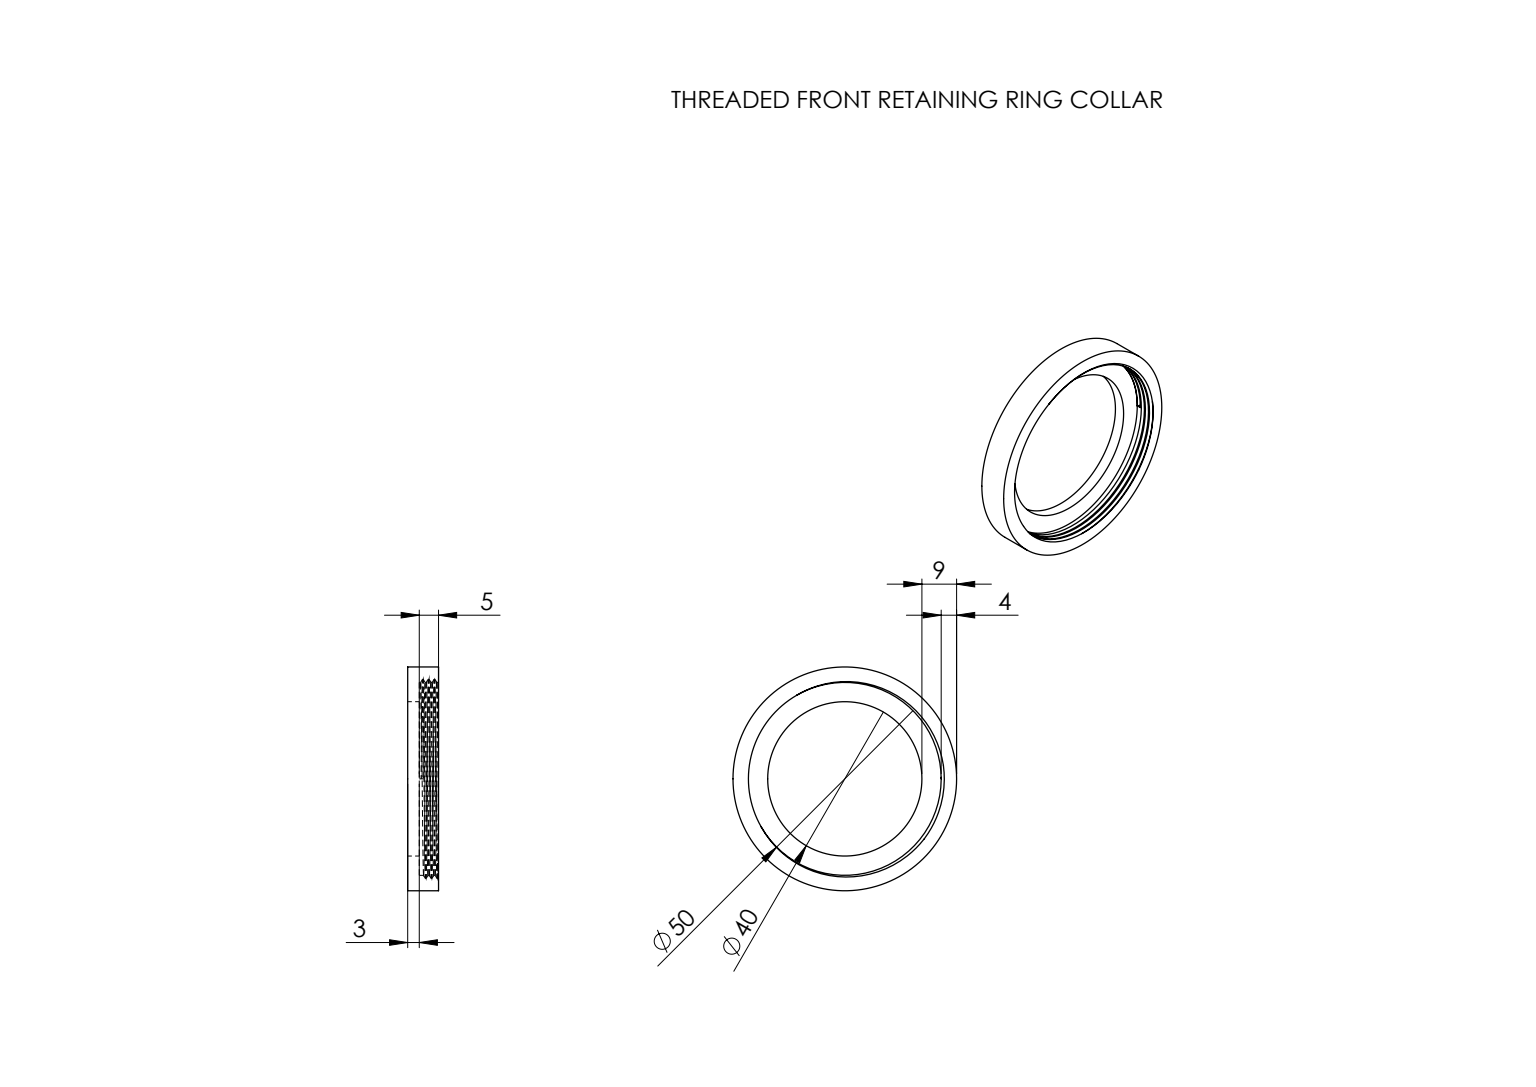
ISO-10303-21;
HEADER;
FILE_DESCRIPTION (('STEP AP214'),
    '1' );
FILE_NAME ('Threaded Front Retaining Ring Collar.step',
    '2026-10-22T10:02:39',
    ( '' ),
    ( '' ),
    'SwSTEP 2.0',
    'SolidWorks 2026',
    '' );
FILE_SCHEMA (( 'AUTOMOTIVE_DESIGN' ));
ENDSEC;

DATA;
#16=CARTESIAN_POINT ( 'NONE',  ( -75.12500000204838102, 44.30836144126050158, -25.81189881249999374 ) ) ;
#42=CARTESIAN_POINT ( 'NONE',  ( -78.87500000204838102, 65.69163855873949842, 25.81189881250000440 ) ) ;
#54=CARTESIAN_POINT ( 'NONE',  ( -72.59375000204838102, 55.00000000000000000, 25.81189881249999729 ) ) ;
#55=EDGE_CURVE ( 'NONE', #2377, #9420, #11722, .T. ) ;
#67=DIRECTION ( 'NONE',  ( -1.000000000000000000, 0.000000000000000000, 0.000000000000000000 ) ) ;
#76=CARTESIAN_POINT ( 'NONE',  ( -72.50000000204839523, 29.18810118750000981, 10.69163855873950020 ) ) ;
#83=ORIENTED_EDGE ( 'NONE', *, *, #6664, .F. ) ;
#110=CARTESIAN_POINT ( 'NONE',  ( -77.75000000204839523, 65.69163855873948421, -25.81189881250000084 ) ) ;
#117=CARTESIAN_POINT ( 'NONE',  ( -78.50000000409677625, 80.00000000000000000, -1.530808498934191324E-15 ) ) ;
#125=AXIS2_PLACEMENT_3D ( 'NONE', #5377, #67, #9915 ) ;
#129=CARTESIAN_POINT ( 'NONE',  ( -79.34375000000000000, 65.35533905932734910, 24.99999999999997158 ) ) ;
#131=VERTEX_POINT ( 'NONE', #8809 ) ;
#166=CARTESIAN_POINT ( 'NONE',  ( -74.56250000204839523, 80.81189881250001861, 10.69163855873948599 ) ) ;
#176=( BOUNDED_CURVE ( )  B_SPLINE_CURVE ( 2, ( #5683, #4899, #11229, #6928, #8370, #6645, #9381, #4776, #5808 ),
 .UNSPECIFIED., .F., .T. ) 
 B_SPLINE_CURVE_WITH_KNOTS ( ( 3, 2, 2, 2, 3 ),
 ( 0.3333333333333335924, 0.3541666666666669627, 0.3750000000000003331, 0.3958333333333336479, 0.4166666666666670182 ),
 .UNSPECIFIED. ) 
 CURVE ( )  GEOMETRIC_REPRESENTATION_ITEM ( )  RATIONAL_B_SPLINE_CURVE ( ( 0.9999999999999990008, 0.9238795325112877377, 1.000000000000000000, 0.9238795325112867385, 1.000000000000000000, 0.9238795325112867385, 1.000000000000000000, 0.9238795325112855172, 1.000000000000001110 ) ) 
 REPRESENTATION_ITEM ( '' )  );
#177=CARTESIAN_POINT ( 'NONE',  ( -75.00000000000000000, 63.49954157109033304, -24.30489545910771909 ) ) ;
#219=CARTESIAN_POINT ( 'NONE',  ( -78.31250000000000000, 72.67766952966368876, -17.67766952966368876 ) ) ;
#225=ORIENTED_EDGE ( 'NONE', *, *, #438, .T. ) ;
#231=CARTESIAN_POINT ( 'NONE',  ( -71.59560441781462714, 80.81189881250000440, 6.916273779317701376 ) ) ;
#238=CARTESIAN_POINT ( 'NONE',  ( -78.87500000204839523, 65.69163855873949842, 25.81189881250000084 ) ) ;
#239=CARTESIAN_POINT ( 'NONE',  ( -75.00000000000002842, 78.51577914341699227, 8.706246595591601078 ) ) ;
#275=CARTESIAN_POINT ( 'NONE',  ( -79.53125000000000000, 80.00000000000001421, 10.35533905932737397 ) ) ;
#288=CARTESIAN_POINT ( 'NONE',  ( -77.93750000204838102, 44.30836144126050158, -25.81189881249999374 ) ) ;
#297=CARTESIAN_POINT ( 'NONE',  ( -75.00000000000000000, 78.71525423744449768, -9.017306879578036671 ) ) ;
#304=CARTESIAN_POINT ( 'NONE',  ( -72.21875000409676204, 65.35533905932737753, 24.99999999999999645 ) ) ;
#307=EDGE_CURVE ( 'NONE', #8475, #1715, #7669, .T. ) ;
#335=CARTESIAN_POINT ( 'NONE',  ( -75.96875000000000000, 30.00000000000001421, 10.35533905932739174 ) ) ;
#347=CARTESIAN_POINT ( 'NONE',  ( -76.81250000204839523, 29.18810118750000981, 10.69163855873950020 ) ) ;
#354=FACE_BOUND ( 'NONE', #1822, .T. ) ;
#361=CARTESIAN_POINT ( 'NONE',  ( -72.12500000409677625, 55.00000000000000000, 24.99999999999999645 ) ) ;
#363=FACE_OUTER_BOUND ( 'NONE', #3792, .T. ) ;
#370=CIRCLE ( 'NONE', #6328, 25.00000000000000355 ) ;
#383=ORIENTED_EDGE ( 'NONE', *, *, #4826, .F. ) ;
#393=VECTOR ( 'NONE', #8335, 1000.000000000000000 ) ;
#397=CARTESIAN_POINT ( 'NONE',  ( -77.37500000000000000, 30.00000000000000355, 4.592425496802573578E-15 ) ) ;
#400=LINE ( 'NONE', #10690, #6493 ) ;
#401=AXIS2_PLACEMENT_3D ( 'NONE', #2687, #9038, #3756 ) ;
#402=CARTESIAN_POINT ( 'NONE',  ( -75.00000000000000000, 55.00000000000000000, 25.00000000000000355 ) ) ;
#410=CARTESIAN_POINT ( 'NONE',  ( -79.06250000204840944, 80.81189881250001861, -10.69163855873949132 ) ) ;
#417=CARTESIAN_POINT ( 'NONE',  ( -79.34375000204839523, 73.25176868561975141, -18.25176868561974430 ) ) ;
#418=PLANE ( 'NONE',  #9121 ) ;
#420=ORIENTED_EDGE ( 'NONE', *, *, #2126, .F. ) ;
#422=CARTESIAN_POINT ( 'NONE',  ( -72.03125000409679046, 44.64466094067262958, 25.00000000000001066 ) ) ;
#438=EDGE_CURVE ( 'NONE', #9864, #879, #4301, .T. ) ;
#451=CARTESIAN_POINT ( 'NONE',  ( -78.87500000000002842, 30.00000000000003553, 4.592425496802568845E-15 ) ) ;
#456=CARTESIAN_POINT ( 'NONE',  ( -72.78125000000002842, 30.00000000000000355, -10.35533905932738108 ) ) ;
#459=DIRECTION ( 'NONE',  ( 1.000000000000000000, -0.000000000000000000, -0.000000000000000000 ) ) ;
#468=CARTESIAN_POINT ( 'NONE',  ( -75.31250000204839523, 29.18810118750000981, 10.69163855873950020 ) ) ;
#475=DIRECTION ( 'NONE',  ( 0.000000000000000000, 0.000000000000000000, 1.000000000000000000 ) ) ;
#478=( GEOMETRIC_REPRESENTATION_CONTEXT ( 3 ) GLOBAL_UNCERTAINTY_ASSIGNED_CONTEXT ( ( #4789 ) ) GLOBAL_UNIT_ASSIGNED_CONTEXT ( ( #10005, #10508, #11461 ) ) REPRESENTATION_CONTEXT ( 'NONE', 'WORKASPACE' ) );
#480=CARTESIAN_POINT ( 'NONE',  ( -79.25000000000000000, 55.00000000000000000, 24.99999999999999645 ) ) ;
#487=CARTESIAN_POINT ( 'NONE',  ( -78.12500000409677625, 55.00000000000000000, 24.99999999999999645 ) ) ;
#510=CARTESIAN_POINT ( 'NONE',  ( -74.18750000000000000, 37.32233047033631124, -17.67766952966368166 ) ) ;
#515=CYLINDRICAL_SURFACE ( 'NONE', #11802, 29.00000000000000355 ) ;
#525=CARTESIAN_POINT ( 'NONE',  ( -76.62500000204839523, 29.18810118750000626, -10.69163855873949309 ) ) ;
#529=CARTESIAN_POINT ( 'NONE',  ( -75.49999999999972999, 55.00000000002793854, -24.99999999999999645 ) ) ;
#532=CARTESIAN_POINT ( 'NONE',  ( -77.84375000204839523, 73.25176868561975141, -18.25176868561974430 ) ) ;
#544=CARTESIAN_POINT ( 'NONE',  ( -78.50000000409677625, 80.00000000000000000, -1.530808498934191324E-15 ) ) ;
#550=CARTESIAN_POINT ( 'NONE',  ( -78.03125000204839523, 36.74823131438024859, -18.25176868561973720 ) ) ;
#557=CARTESIAN_POINT ( 'NONE',  ( -75.00000000000004263, 38.53867536077979139, -19.88773376194887987 ) ) ;
#559=ORIENTED_EDGE ( 'NONE', *, *, #6186, .F. ) ;
#566=AXIS2_PLACEMENT_3D ( 'NONE', #8644, #10369, #4811 ) ;
#568=CARTESIAN_POINT ( 'NONE',  ( -73.25000000000000000, 55.00000000000000000, 24.99999999999999645 ) ) ;
#582=CARTESIAN_POINT ( 'NONE',  ( -73.15625000204839523, 73.25176868561975141, -18.25176868561974430 ) ) ;
#601=ORIENTED_EDGE ( 'NONE', *, *, #9027, .F. ) ;
#614=CARTESIAN_POINT ( 'NONE',  ( -76.62500000204839523, 29.18810118750000626, -10.69163855873949309 ) ) ;
#618=CARTESIAN_POINT ( 'NONE',  ( -74.99999999999997158, 37.75762616273102168, -19.19216994046665903 ) ) ;
#627=CARTESIAN_POINT ( 'NONE',  ( -73.90625000000001421, 65.35533905932737753, -24.99999999999999645 ) ) ;
#629=ADVANCED_FACE ( 'NONE', ( #7359 ), #4594, .T. ) ;
#638=DIRECTION ( 'NONE',  ( -1.000000000000000000, 0.000000000000000000, 0.000000000000000000 ) ) ;
#641=CARTESIAN_POINT ( 'NONE',  ( -74.93750000204839523, 44.30836144126050158, -25.81189881249999374 ) ) ;
#649=CARTESIAN_POINT ( 'NONE',  ( -75.87500000204838102, 65.69163855873949842, 25.81189881250000084 ) ) ;
#667=CARTESIAN_POINT ( 'NONE',  ( -74.84375000204839523, 55.00000000000000000, -25.81189881249999729 ) ) ;
#674=CARTESIAN_POINT ( 'NONE',  ( -74.99999999999998579, 36.28446816562487243, -17.71219965803775764 ) ) ;
#675=ORIENTED_EDGE ( 'NONE', *, *, #799, .F. ) ;
#685=CARTESIAN_POINT ( 'NONE',  ( -71.95822497812569907, 74.53807824654330716, 16.15905817987090032 ) ) ;
#689=CARTESIAN_POINT ( 'NONE',  ( -80.00000000000000000, 55.00000000000000000, -24.99999999999999645 ) ) ;
#693=VECTOR ( 'NONE', #6124, 1000.000000000000000 ) ;
#694=CARTESIAN_POINT ( 'NONE',  ( -74.99999999999998579, 39.36515909056227258, -20.53791299142420712 ) ) ;
#705=CARTESIAN_POINT ( 'NONE',  ( -75.03125000204838102, 55.00000000000000000, -25.81189881249999729 ) ) ;
#725=CARTESIAN_POINT ( 'NONE',  ( -78.50000000204840944, 44.30836144126053000, 25.81189881250000795 ) ) ;
#728=CARTESIAN_POINT ( 'NONE',  ( -76.62500000409677625, 55.00000000000000000, 24.99999999999999645 ) ) ;
#730=CARTESIAN_POINT ( 'NONE',  ( -75.00000000000001421, 29.55542218757419803, 0.4186910811744771199 ) ) ;
#742=CARTESIAN_POINT ( 'NONE',  ( -72.40625000204838102, 29.18810118750000271, 4.741568889096522788E-15 ) ) ;
#748=VECTOR ( 'NONE', #2550, 1000.000000000000000 ) ;
#763=B_SPLINE_CURVE_WITH_KNOTS ( 'NONE', 3,
 ( #2945, #11252, #6612, #5710, #177, #2885, #3718, #10057, #10117, #6673, #7383, #6488, #10302, #1917, #5585, #3779, #4804, #9408, #8461, #10239, #1201, #8516, #297, #9170, #4743, #9347, #4678, #1016, #7622, #1855, #6554, #1135, #8329, #7448, #10183, #239, #9282, #1319, #3124, #9702 ),
 .UNSPECIFIED., .F., .F.,
 ( 4, 2, 2, 2, 2, 2, 2, 2, 2, 2, 2, 2, 2, 2, 2, 2, 2, 2, 2, 4 ),
 ( 2.472710646779110686E-15, 0.003130555644250782206, 0.006261111288499070747, 0.009391666932747358421, 0.01095694475487150529, 0.01252222257699565390, 0.01565277822124398407, 0.01721805604336814829, 0.01878333386549230904, 0.02504444515398900756, 0.02660972297611319259, 0.02817500079823737763, 0.03130555644248574770, 0.03443611208673411084, 0.03600138990885830281, 0.03756666773098249479, 0.04382777901947923493, 0.04539305684160341997, 0.04695833466372760501, 0.05008889030797599590 ),
 .UNSPECIFIED. ) ;
#769=CARTESIAN_POINT ( 'NONE',  ( -74.84375000204839523, 73.25176868561975141, -18.25176868561974430 ) ) ;
#784=CARTESIAN_POINT ( 'NONE',  ( -76.06250000204840944, 80.81189881250001861, -10.69163855873949132 ) ) ;
#790=CARTESIAN_POINT ( 'NONE',  ( -75.00000000000000000, 34.71505921034813724, 14.90932262158721500 ) ) ;
#799=EDGE_CURVE ( 'NONE', #1715, #10833, #3542, .T. ) ;
#801=CARTESIAN_POINT ( 'NONE',  ( -72.68750000204839523, 44.30836144126053000, 25.81189881250000795 ) ) ;
#823=CARTESIAN_POINT ( 'NONE',  ( -83.00000000000000000, 55.00000000000000000, 20.00000000000000355 ) ) ;
#832=CARTESIAN_POINT ( 'NONE',  ( -76.53125000204839523, 36.74823131438024859, -18.25176868561973720 ) ) ;
#838=CARTESIAN_POINT ( 'NONE',  ( -75.59375000409679046, 80.00000000000001421, -10.35533905932737753 ) ) ;
#855=CARTESIAN_POINT ( 'NONE',  ( -75.03125000204838102, 55.00000000000000000, -25.81189881249999729 ) ) ;
#870=ORIENTED_EDGE ( 'NONE', *, *, #7718, .F. ) ;
#879=VERTEX_POINT ( 'NONE', #5025 ) ;
#891=CARTESIAN_POINT ( 'NONE',  ( -76.62500000204838102, 29.18810118750000626, -10.69163855873949132 ) ) ;
#897=CARTESIAN_POINT ( 'NONE',  ( -76.62500000409677625, 55.00000000000000000, 24.99999999999999645 ) ) ;
#898=CARTESIAN_POINT ( 'NONE',  ( -75.50000000409677625, 80.00000000000000000, -1.530808498934191324E-15 ) ) ;
#906=ORIENTED_EDGE ( 'NONE', *, *, #8266, .F. ) ;
#912=MANIFOLD_SOLID_BREP ( 'Cavity1', #11314 ) ;
#913=EDGE_CURVE ( 'NONE', #1407, #8886, #6011, .T. ) ;
#914=CARTESIAN_POINT ( 'NONE',  ( -74.18750000204838102, 44.30836144126053000, 25.81189881250000795 ) ) ;
#924=AXIS2_PLACEMENT_3D ( 'NONE', #3401, #7187, #2623 ) ;
#936=AXIS2_PLACEMENT_3D ( 'NONE', #10985, #6463, #1890 ) ;
#945=CARTESIAN_POINT ( 'NONE',  ( -76.71875000204839523, 36.74823131438024859, -18.25176868561973720 ) ) ;
#953=CARTESIAN_POINT ( 'NONE',  ( -75.00000000000000000, 55.00000000000000000, 29.00000000000000355 ) ) ;
#958=DIRECTION ( 'NONE',  ( 0.000000000000000000, 0.000000000000000000, -1.000000000000000000 ) ) ;
#963=CARTESIAN_POINT ( 'NONE',  ( -73.25000000204839523, 65.69163855873948421, -25.81189881250000440 ) ) ;
#981=CARTESIAN_POINT ( 'NONE',  ( -72.31250000204839523, 29.18810118750000626, -10.69163855873949309 ) ) ;
#1006=CARTESIAN_POINT ( 'NONE',  ( -83.00000000000000000, 55.00000000000000000, 29.00000000000000355 ) ) ;
#1009=CARTESIAN_POINT ( 'NONE',  ( -76.43750000204838102, 65.69163855873948421, -25.81189881250000440 ) ) ;
#1014=CARTESIAN_POINT ( 'NONE',  ( -78.96875000204839523, 80.81189881250000440, -1.580522963032174394E-15 ) ) ;
#1016=CARTESIAN_POINT ( 'NONE',  ( -75.00000000000001421, 80.17654715216286831, -1.959916203278639024 ) ) ;
#1020=CARTESIAN_POINT ( 'NONE',  ( -71.56250000204838102, 80.81189881250001861, -10.69163855873949132 ) ) ;
#1067=CARTESIAN_POINT ( 'NONE',  ( -73.25000000204838102, 80.81189881250001861, -10.69163855873949132 ) ) ;
#1080=VECTOR ( 'NONE', #11683, 1000.000000000000000 ) ;
#1082=CARTESIAN_POINT ( 'NONE',  ( -76.53125000409677625, 44.64466094067262958, 25.00000000000001066 ) ) ;
#1104=CARTESIAN_POINT ( 'NONE',  ( -80.00000000000000000, 55.00000000000000000, -24.99999999999999645 ) ) ;
#1115=CARTESIAN_POINT ( 'NONE',  ( -79.62500000000000000, 80.00000000000000000, -1.530808498934191324E-15 ) ) ;
#1127=CARTESIAN_POINT ( 'NONE',  ( -73.71875000204839523, 36.74823131438024859, -18.25176868561973720 ) ) ;
#1134=CARTESIAN_POINT ( 'NONE',  ( -79.53125000204838102, 55.00000000000000000, -25.81189881249999729 ) ) ;
#1135=CARTESIAN_POINT ( 'NONE',  ( -75.00000000000001421, 80.11351121041060708, 2.705448568323045144 ) ) ;
#1140=CARTESIAN_POINT ( 'NONE',  ( -73.53125000409676204, 44.64466094067262958, 25.00000000000001066 ) ) ;
#1178=CARTESIAN_POINT ( 'NONE',  ( -78.21875000000001421, 80.00000000000001421, -10.35533905932737753 ) ) ;
#1194=CARTESIAN_POINT ( 'NONE',  ( -79.15625000204839523, 73.25176868561975141, -18.25176868561974430 ) ) ;
#1201=CARTESIAN_POINT ( 'NONE',  ( -75.00000000000000000, 78.13883143010173171, -10.47133000126702917 ) ) ;
#1205=CARTESIAN_POINT ( 'NONE',  ( -74.18750000409677625, 72.67766952966368876, -17.67766952966368876 ) ) ;
#1223=CARTESIAN_POINT ( 'NONE',  ( -78.12500000000004263, 79.99999999999992895, -1.530808498934187183E-15 ) ) ;
#1228=CARTESIAN_POINT ( 'NONE',  ( -78.50000000000000000, 55.00000000000000000, -24.99999999999999645 ) ) ;
#1231=CARTESIAN_POINT ( 'NONE',  ( -75.00000000000001421, 76.68791387293471473, 12.43520775219157315 ) ) ;
#1233=CARTESIAN_POINT ( 'NONE',  ( -79.06250000000001421, 37.32233047033631124, 17.67766952966369232 ) ) ;
#1234=CARTESIAN_POINT ( 'NONE',  ( -74.99999999999997158, 42.18634379380805655, -22.42280631998790597 ) ) ;
#1237=FACE_OUTER_BOUND ( 'NONE', #7141, .T. ) ;
#1246=CARTESIAN_POINT ( 'NONE',  ( -77.18750000204839523, 65.69163855873949842, 25.81189881250000440 ) ) ;
#1260=CARTESIAN_POINT ( 'NONE',  ( -74.65625000409679046, 30.00000000000000355, -10.35533905932738108 ) ) ;
#1273=ORIENTED_EDGE ( 'NONE', *, *, #5965, .F. ) ;
#1274=EDGE_CURVE ( 'NONE', #2004, #9652, #8220, .T. ) ;
#1296=ORIENTED_EDGE ( 'NONE', *, *, #9433, .T. ) ;
#1297=CARTESIAN_POINT ( 'NONE',  ( -76.62500000000000000, 80.00000000000000000, -1.530808498934191324E-15 ) ) ;
#1306=ADVANCED_FACE ( 'NONE', ( #9805 ), #10699, .F. ) ;
#1311=CARTESIAN_POINT ( 'NONE',  ( -72.78125000204838102, 55.00000000000000000, 25.81189881249999729 ) ) ;
#1319=CARTESIAN_POINT ( 'NONE',  ( -74.99999999999997158, 77.69762738690542392, 10.61382896765898209 ) ) ;
#1321=EDGE_CURVE ( 'NONE', #10439, #8197, #10496, .T. ) ;
#1327=CARTESIAN_POINT ( 'NONE',  ( -74.00000000409677625, 80.00000000000000000, -1.530808498934191324E-15 ) ) ;
#1336=CARTESIAN_POINT ( 'NONE',  ( -75.87500000409677625, 55.00000000000000000, -24.99999999999999645 ) ) ;
#1340=B_SPLINE_CURVE_WITH_KNOTS ( 'NONE', 3,
 ( #4066, #4114, #7773, #1234, #11351, #11403, #3216, #8729, #4903, #6884, #2982, #10281, #5750, #9385, #8555 ),
 .UNSPECIFIED., .F., .F.,
 ( 4, 2, 1, 2, 2, 2, 2, 4 ),
 ( 2.418898813002652444E-15, 0.002548748984084002640, 0.005097497968165586209, 0.007646246952247169777, 0.01019499593632875248, 0.01529249390449191962, 0.01784124288857351706, 0.02038999187265511104 ),
 .UNSPECIFIED. ) ;
#1360=ORIENTED_EDGE ( 'NONE', *, *, #1799, .T. ) ;
#1361=CARTESIAN_POINT ( 'NONE',  ( -74.00000000000000000, 55.00000000000000000, -24.99999999999999645 ) ) ;
#1376=CARTESIAN_POINT ( 'NONE',  ( -72.50000000204839523, 44.30836144126053000, 25.81189881250000795 ) ) ;
#1383=DIRECTION ( 'NONE',  ( 1.000000000000000000, 0.000000000000000000, 0.000000000000000000 ) ) ;
#1391=CARTESIAN_POINT ( 'NONE',  ( -72.59375000409677625, 80.00000000000001421, -10.35533905932737753 ) ) ;
#1401=FACE_OUTER_BOUND ( 'NONE', #8358, .T. ) ;
#1407=VERTEX_POINT ( 'NONE', #3518 ) ;
#1411=( BOUNDED_SURFACE ( )  B_SPLINE_SURFACE ( 1, 2, ( 
 ( #9364, #7103, #10667, #8770, #1629, #6085, #3316, #8950, #7878, #725, #1514, #10729, #11566, #5178, #550, #4458, #6984, #4215, #1459, #6204, #11509, #3369, #10605, #2412, #9838, #9718, #8888, #2538, #8049, #614, #2596, #8111, #8833, #9661, #7046, #784, #2477, #11746, #4276, #6142, #9779, #5355, #5296, #7934, #6027, #1575, #7161, #5240, #667, #11691, #4338, #7988, #3430, #11627, #4398, #3495, #10785, #6264, #9895, #5123, #1689, #6927, #9006, #10557, #2357, #963, #10063, #3723, #5596, #10960, #9233, #7222, #54, #6431, #4682, #10907, #7452, #6560, #5526, #11080, #7277, #2826, #8279, #1020, #6492, #7387, #8334 ),
 ( #4571, #9952, #3550, #3610, #117, #1861, #3784, #8225, #9176, #4628, #2717, #1923, #10122, #2770, #5468, #2891, #6379, #10190, #11014, #4509, #1800, #1980, #10006, #5649, #9287, #1082, #9116, #4748, #8399, #10849, #2654, #6321, #1750, #5413, #9061, #838, #898, #8164, #11806, #2394, #3670, #7334, #8521, #9474, #6678, #1260, #9413, #11257, #6795, #10306, #1205, #10244, #1327, #4930, #6857, #2164, #3184, #1140, #3128, #5777, #3907, #4870, #10423, #5834, #9351, #2104, #3069, #1391, #2224, #5892, #3968, #304, #361, #422, #7515, #11136, #9535, #6616, #4028, #2041, #7571, #4084, #10481, #8586, #7744, #11198, #11320 ) ),
 .UNSPECIFIED., .F., .F., .T. ) 
 B_SPLINE_SURFACE_WITH_KNOTS ( ( 2, 2 ),
 ( 3, 2, 2, 2, 2, 2, 2, 2, 2, 2, 2, 2, 2, 2, 2, 2, 2, 2, 2, 2, 2, 2, 2, 2, 2, 2, 2, 2, 2, 2, 2, 2, 2, 2, 2, 2, 2, 2, 2, 2, 2, 2, 2, 3 ),
 ( 0.000000000000000000, 1.000000000000000000 ),
 ( 0.000000000000000000, 0.02083333333333333218, 0.04166666666666666435, 0.06250000000000000000, 0.08333333333333332871, 0.1041666666666666713, 0.1250000000000000000, 0.1458333333333333426, 0.1666666666666666574, 0.1875000000000000000, 0.2083333333333333426, 0.2291666666666666574, 0.2500000000000000000, 0.2708333333333333148, 0.2916666666666666852, 0.3125000000000000000, 0.3333333333333333148, 0.3541666666666666852, 0.3750000000000000000, 0.3958333333333333148, 0.4166666666666666852, 0.4375000000000000000, 0.4583333333333333148, 0.4791666666666666852, 0.5000000000000000000, 0.5208333333333333703, 0.5416666666666666297, 0.5625000000000000000, 0.5833333333333333703, 0.6041666666666666297, 0.6250000000000000000, 0.6458333333333333703, 0.6666666666666666297, 0.6875000000000000000, 0.7083333333333333703, 0.7291666666666666297, 0.7500000000000000000, 0.7708333333333333703, 0.7916666666666666297, 0.8125000000000000000, 0.8333333333333333703, 0.8541666666666666297, 0.8750000000000000000, 0.8888490476107191451 ),
 .UNSPECIFIED. ) 
 GEOMETRIC_REPRESENTATION_ITEM ( )  RATIONAL_B_SPLINE_SURFACE ( (
 ( 1.000000000000000000, 0.9238795325112867385, 1.000000000000000000, 0.9238795325112867385, 1.000000000000000000, 0.9238795325112867385, 1.000000000000000000, 0.9238795325112867385, 1.000000000000000000, 0.9238795325112867385, 1.000000000000000000, 0.9238795325112867385, 1.000000000000000000, 0.9238795325112867385, 1.000000000000000000, 0.9238795325112867385, 1.000000000000000000, 0.9238795325112867385, 1.000000000000000000, 0.9238795325112867385, 1.000000000000000000, 0.9238795325112867385, 1.000000000000000000, 0.9238795325112867385, 1.000000000000000000, 0.9238795325112867385, 1.000000000000000000, 0.9238795325112867385, 1.000000000000000000, 0.9238795325112867385, 1.000000000000000000, 0.9238795325112867385, 1.000000000000000000, 0.9238795325112867385, 1.000000000000000000, 0.9238795325112867385, 1.000000000000000000, 0.9238795325112867385, 1.000000000000000000, 0.9238795325112867385, 1.000000000000000000, 0.9238795325112867385, 1.000000000000000000, 0.9238795325112867385, 1.000000000000000000, 0.9238795325112867385, 1.000000000000000000, 0.9238795325112867385, 1.000000000000000000, 0.9238795325112867385, 1.000000000000000000, 0.9238795325112867385, 1.000000000000000000, 0.9238795325112867385, 1.000000000000000000, 0.9238795325112867385, 1.000000000000000000, 0.9238795325112867385, 1.000000000000000000, 0.9238795325112867385, 1.000000000000000000, 0.9238795325112867385, 1.000000000000000000, 0.9238795325112867385, 1.000000000000000000, 0.9238795325112867385, 1.000000000000000000, 0.9238795325112867385, 1.000000000000000000, 0.9238795325112867385, 1.000000000000000000, 0.9238795325112867385, 1.000000000000000000, 0.9238795325112867385, 1.000000000000000000, 0.9238795325112867385, 1.000000000000000000, 0.9238795325112867385, 1.000000000000000000, 0.9238795325112867385, 1.000000000000000000, 0.9238795325112867385, 1.000000000000000000, 0.9238795325112867385, 1.000000000000000000, 0.9493985930367334625, 0.9660721903170175207),
 ( 1.000000000000000000, 0.9238795325112867385, 1.000000000000000000, 0.9238795325112867385, 1.000000000000000000, 0.9238795325112867385, 1.000000000000000000, 0.9238795325112867385, 1.000000000000000000, 0.9238795325112867385, 1.000000000000000000, 0.9238795325112867385, 1.000000000000000000, 0.9238795325112867385, 1.000000000000000000, 0.9238795325112867385, 1.000000000000000000, 0.9238795325112867385, 1.000000000000000000, 0.9238795325112867385, 1.000000000000000000, 0.9238795325112867385, 1.000000000000000000, 0.9238795325112867385, 1.000000000000000000, 0.9238795325112867385, 1.000000000000000000, 0.9238795325112867385, 1.000000000000000000, 0.9238795325112867385, 1.000000000000000000, 0.9238795325112867385, 1.000000000000000000, 0.9238795325112867385, 1.000000000000000000, 0.9238795325112867385, 1.000000000000000000, 0.9238795325112867385, 1.000000000000000000, 0.9238795325112867385, 1.000000000000000000, 0.9238795325112867385, 1.000000000000000000, 0.9238795325112867385, 1.000000000000000000, 0.9238795325112867385, 1.000000000000000000, 0.9238795325112867385, 1.000000000000000000, 0.9238795325112867385, 1.000000000000000000, 0.9238795325112867385, 1.000000000000000000, 0.9238795325112867385, 1.000000000000000000, 0.9238795325112867385, 1.000000000000000000, 0.9238795325112867385, 1.000000000000000000, 0.9238795325112867385, 1.000000000000000000, 0.9238795325112867385, 1.000000000000000000, 0.9238795325112867385, 1.000000000000000000, 0.9238795325112867385, 1.000000000000000000, 0.9238795325112867385, 1.000000000000000000, 0.9238795325112867385, 1.000000000000000000, 0.9238795325112867385, 1.000000000000000000, 0.9238795325112867385, 1.000000000000000000, 0.9238795325112867385, 1.000000000000000000, 0.9238795325112867385, 1.000000000000000000, 0.9238795325112867385, 1.000000000000000000, 0.9238795325112867385, 1.000000000000000000, 0.9238795325112867385, 1.000000000000000000, 0.9493985930367334625, 0.9660721903170175207) ) ) 
 REPRESENTATION_ITEM ( '' )  SURFACE ( )  );
#1416=DIRECTION ( 'NONE',  ( 0.000000000000000000, 0.000000000000000000, 1.000000000000000000 ) ) ;
#1418=CARTESIAN_POINT ( 'NONE',  ( -78.12500000409677625, 55.00000000000000000, 24.99999999999999645 ) ) ;
#1420=CARTESIAN_POINT ( 'NONE',  ( -72.31250000000000000, 72.67766952966368876, -17.67766952966368876 ) ) ;
#1432=CARTESIAN_POINT ( 'NONE',  ( -75.12500000204838102, 29.18810118750000626, -10.69163855873949309 ) ) ;
#1450=CARTESIAN_POINT ( 'NONE',  ( -77.75000000000000000, 55.00000000000000000, 24.99999999999999645 ) ) ;
#1459=CARTESIAN_POINT ( 'NONE',  ( -77.65625000204839523, 73.25176868561975141, -18.25176868561974430 ) ) ;
#1466=CARTESIAN_POINT ( 'NONE',  ( -75.00000000000004263, 33.65755212260173579, -14.43688233189822334 ) ) ;
#1470=EDGE_LOOP ( 'NONE', ( #2824, #11364, #11751, #8308 ) ) ;
#1477=CARTESIAN_POINT ( 'NONE',  ( -77.75000000204839523, 80.81189881250001861, -10.69163855873949132 ) ) ;
#1479=( BOUNDED_CURVE ( )  B_SPLINE_CURVE ( 2, ( #8361, #5801, #5616, #9435, #1223, #10269, #5552, #7412, #10146 ),
 .UNSPECIFIED., .F., .T. ) 
 B_SPLINE_CURVE_WITH_KNOTS ( ( 3, 2, 2, 2, 3 ),
 ( 0.1584082455038353654, 0.1782132311131151281, 0.1980182167223948908, 0.2178232023316745980, 0.2376281879409543607 ),
 .UNSPECIFIED. ) 
 CURVE ( )  GEOMETRIC_REPRESENTATION_ITEM ( )  RATIONAL_B_SPLINE_CURVE ( ( 1.000000000000020650, 0.9238795325112661994, 1.000000000000000000, 0.9238795325112868495, 1.000000000000000000, 0.9238795325112868495, 1.000000000000000000, 0.9238795325112363344, 1.000000000000050404 ) ) 
 REPRESENTATION_ITEM ( '' )  );
#1485=EDGE_CURVE ( 'NONE', #4583, #10943, #11068, .T. ) ;
#1491=CARTESIAN_POINT ( 'NONE',  ( -73.62500000204842365, 29.18810118750000626, -10.69163855873949309 ) ) ;
#1498=CARTESIAN_POINT ( 'NONE',  ( -76.53125000204838102, 55.00000000000000000, -25.81189881249999729 ) ) ;
#1509=CARTESIAN_POINT ( 'NONE',  ( -77.09375000000004263, 44.64466094067264379, -24.99999999999989697 ) ) ;
#1514=CARTESIAN_POINT ( 'NONE',  ( -78.40625000204839523, 36.74823131438026280, 18.25176868561974786 ) ) ;
#1532=CARTESIAN_POINT ( 'NONE',  ( -78.96875000204839523, 73.25176868561975141, 18.25176868561974075 ) ) ;
#1545=CARTESIAN_POINT ( 'NONE',  ( -73.34375000204839523, 55.00000000000000000, -25.81189881249999729 ) ) ;
#1555=CARTESIAN_POINT ( 'NONE',  ( -75.31250000204839523, 29.18810118750000626, -10.69163855873949132 ) ) ;
#1575=CARTESIAN_POINT ( 'NONE',  ( -75.12500000204838102, 29.18810118750000626, -10.69163855873949309 ) ) ;
#1579=CARTESIAN_POINT ( 'NONE',  ( -74.99999999999998579, 36.75304232195939136, 17.29401847480263754 ) ) ;
#1580=EDGE_LOOP ( 'NONE', ( #1273, #4112 ) ) ;
#1588=CARTESIAN_POINT ( 'NONE',  ( -76.81250000204838102, 29.18810118750000626, -10.69163855873949309 ) ) ;
#1629=CARTESIAN_POINT ( 'NONE',  ( -78.96875000204839523, 80.81189881250000440, -1.580522963032174394E-15 ) ) ;
#1633=CARTESIAN_POINT ( 'NONE',  ( -74.99999999999992895, 32.96633592742742991, 12.31671744011198122 ) ) ;
#1636=APPLICATION_CONTEXT ( 'automotive_design' ) ;
#1643=CARTESIAN_POINT ( 'NONE',  ( -73.34375000204839523, 73.25176868561975141, -18.25176868561974430 ) ) ;
#1646=( NAMED_UNIT ( * ) PLANE_ANGLE_UNIT ( ) SI_UNIT ( $, .RADIAN. ) );
#1657=DIRECTION ( 'NONE',  ( 0.000000000000000000, 0.000000000000000000, 1.000000000000000000 ) ) ;
#1660=CARTESIAN_POINT ( 'NONE',  ( -77.00000000000000000, 55.00000000000000000, -24.99999999999999645 ) ) ;
#1668=EDGE_CURVE ( 'NONE', #10082, #7521, #3824, .T. ) ;
#1686=PLANE ( 'NONE',  #11039 ) ;
#1689=CARTESIAN_POINT ( 'NONE',  ( -73.71875000204839523, 29.18810118750000271, 4.741568889096522788E-15 ) ) ;
#1697=CARTESIAN_POINT ( 'NONE',  ( -75.00000000000000000, 30.81391793133463608, -8.312227262611900258 ) ) ;
#1707=CARTESIAN_POINT ( 'NONE',  ( -74.28125000204838102, 55.00000000000000000, 25.81189881249999729 ) ) ;
#1715=VERTEX_POINT ( 'NONE', #1418 ) ;
#1736=CARTESIAN_POINT ( 'NONE',  ( -78.68750000204838102, 44.30836144126053000, 25.81189881250000795 ) ) ;
#1743=CARTESIAN_POINT ( 'NONE',  ( -76.43750000204839523, 44.30836144126049447, -25.81189881249999019 ) ) ;
#1744=LINE ( 'NONE', #6258, #1080 ) ;
#1748=PRODUCT ( 'Threaded Front Retaining Ring Collar', 'Threaded Front Retaining Ring Collar', '', ( #7457 ) ) ;
#1750=CARTESIAN_POINT ( 'NONE',  ( -75.87500000409677625, 55.00000000000000000, -24.99999999999999645 ) ) ;
#1777=CARTESIAN_POINT ( 'NONE',  ( -75.00000000000000000, 55.00000000000000000, 29.00000000000000355 ) ) ;
#1789=CARTESIAN_POINT ( 'NONE',  ( -77.28125000204838102, 55.00000000000000000, 25.81189881249999729 ) ) ;
#1795=CARTESIAN_POINT ( 'NONE',  ( -74.99999999999998579, 39.36515909056227258, -20.53791299142421067 ) ) ;
#1799=EDGE_CURVE ( 'NONE', #5071, #8389, #2191, .T. ) ;
#1800=CARTESIAN_POINT ( 'NONE',  ( -77.00000000409677625, 80.00000000000000000, -1.530808498934191324E-15 ) ) ;
#1814=CARTESIAN_POINT ( 'NONE',  ( -75.31250000204839523, 29.18810118750000626, -10.69163855873949309 ) ) ;
#1819=ADVANCED_FACE ( 'NONE', ( #9566 ), #7720, .F. ) ;
#1822=EDGE_LOOP ( 'NONE', ( #6558, #2902 ) ) ;
#1846=CARTESIAN_POINT ( 'NONE',  ( -75.68750000204838102, 44.30836144126053000, 25.81189881250000795 ) ) ;
#1854=CARTESIAN_POINT ( 'NONE',  ( -79.34375000204839523, 55.00000000000000000, -25.81189881249999729 ) ) ;
#1855=CARTESIAN_POINT ( 'NONE',  ( -75.00000000000000000, 80.22492272376648259, -0.3963795942728437494 ) ) ;
#1861=CARTESIAN_POINT ( 'NONE',  ( -78.40625000409677625, 80.00000000000001421, 10.35533905932737397 ) ) ;
#1875=CARTESIAN_POINT ( 'NONE',  ( -72.12500000204839523, 44.30836144126050158, -25.81189881249999374 ) ) ;
#1890=DIRECTION ( 'NONE',  ( 0.000000000000000000, 0.000000000000000000, 1.000000000000000000 ) ) ;
#1891=DIRECTION ( 'NONE',  ( -1.000000000000000000, 0.000000000000000000, 0.000000000000000000 ) ) ;
#1908=AXIS2_PLACEMENT_3D ( 'NONE', #4429, #10814, #3638 ) ;
#1917=CARTESIAN_POINT ( 'NONE',  ( -75.00000000000001421, 72.60765915417964322, -18.52300487688723152 ) ) ;
#1923=CARTESIAN_POINT ( 'NONE',  ( -77.84375000409677625, 30.00000000000001421, 10.35533905932739174 ) ) ;
#1932=CARTESIAN_POINT ( 'NONE',  ( -79.62500000000001421, 79.99999999999997158, -1.530808498934189944E-15 ) ) ;
#1944=ORIENTED_EDGE ( 'NONE', *, *, #6664, .T. ) ;
#1969=CARTESIAN_POINT ( 'NONE',  ( -77.65625000204839523, 73.25176868561975141, -18.25176868561974430 ) ) ;
#1978=ORIENTED_EDGE ( 'NONE', *, *, #7125, .F. ) ;
#1980=CARTESIAN_POINT ( 'NONE',  ( -76.90625000409677625, 80.00000000000001421, 10.35533905932737397 ) ) ;
#1988=FACE_OUTER_BOUND ( 'NONE', #5112, .T. ) ;
#1991=CARTESIAN_POINT ( 'NONE',  ( -79.53125000000001421, 79.99999999999998579, 10.35533905932735799 ) ) ;
#1993=EDGE_LOOP ( 'NONE', ( #1978, #9827, #1296, #10861 ) ) ;
#2004=VERTEX_POINT ( 'NONE', #1006 ) ;
#2008=CARTESIAN_POINT ( 'NONE',  ( -77.65625000409676204, 30.00000000000000355, -10.35533905932738108 ) ) ;
#2012=CARTESIAN_POINT ( 'NONE',  ( -76.06250000000000000, 37.32233047033631124, 17.67766952966369232 ) ) ;
#2026=CARTESIAN_POINT ( 'NONE',  ( -72.03125000204838102, 55.00000000000000000, -25.81189881249999729 ) ) ;
#2041=CARTESIAN_POINT ( 'NONE',  ( -71.46875000409677625, 44.64466094067260826, -24.99999999999998934 ) ) ;
#2050=( GEOMETRIC_REPRESENTATION_CONTEXT ( 3 ) GLOBAL_UNCERTAINTY_ASSIGNED_CONTEXT ( ( #2479 ) ) GLOBAL_UNIT_ASSIGNED_CONTEXT ( ( #11367, #1646, #5315 ) ) REPRESENTATION_CONTEXT ( 'NONE', 'WORKASPACE' ) );
#2060=EDGE_CURVE ( 'NONE', #5404, #8475, #1479, .T. ) ;
#2067=CARTESIAN_POINT ( 'NONE',  ( -75.00000000000000000, 55.00000000000000000, 0.000000000000000000 ) ) ;
#2071=CARTESIAN_POINT ( 'NONE',  ( -78.03125000409679046, 44.64466094067260826, 24.99999999999998579 ) ) ;
#2075=CARTESIAN_POINT ( 'NONE',  ( -75.12500000000000000, 80.00000000000000000, -1.530808498934191324E-15 ) ) ;
#2088=CARTESIAN_POINT ( 'NONE',  ( -78.21875000204839523, 29.18810118750000271, 4.741568889096522788E-15 ) ) ;
#2096=CARTESIAN_POINT ( 'NONE',  ( -79.43750000204838102, 65.69163855873948421, -25.81189881250000084 ) ) ;
#2097=ADVANCED_FACE ( 'NONE', ( #9255 ), #4648, .F. ) ;
#2104=CARTESIAN_POINT ( 'NONE',  ( -72.78125000409679046, 65.35533905932737753, -24.99999999999999645 ) ) ;
#2126=EDGE_CURVE ( 'NONE', #10943, #5071, #8484, .T. ) ;
#2128=DIRECTION ( 'NONE',  ( 0.000000000000000000, 0.000000000000000000, 1.000000000000000000 ) ) ;
#2134=CARTESIAN_POINT ( 'NONE',  ( -75.00000000000000000, 55.00000000000000000, 0.000000000000000000 ) ) ;
#2136=DIRECTION ( 'NONE',  ( 0.000000000000000000, 0.000000000000000000, 1.000000000000000000 ) ) ;
#2140=CARTESIAN_POINT ( 'NONE',  ( -74.84375000000000000, 65.35533905932737753, 24.99999999999999645 ) ) ;
#2152=CARTESIAN_POINT ( 'NONE',  ( -74.00000000204839523, 29.18810118750000981, 10.69163855873950020 ) ) ;
#2164=CARTESIAN_POINT ( 'NONE',  ( -73.71875000409677625, 65.35533905932737753, 24.99999999999999645 ) ) ;
#2191=LINE ( 'NONE', #9623, #7470 ) ;
#2196=( BOUNDED_CURVE ( )  B_SPLINE_CURVE ( 2, ( #7999, #4161, #10613 ),
 .UNSPECIFIED., .F., .T. ) 
 B_SPLINE_CURVE_WITH_KNOTS ( ( 3, 3 ),
 ( 0.4166666666666670182, 0.4304371013617913633 ),
 .UNSPECIFIED. ) 
 CURVE ( )  GEOMETRIC_REPRESENTATION_ITEM ( )  RATIONAL_B_SPLINE_CURVE ( ( 0.9999999999999987788, 0.9496858275272472838, 0.9658850655769216642 ) ) 
 REPRESENTATION_ITEM ( '' )  );
#2202=DIRECTION ( 'NONE',  ( -1.000000000000000000, 0.000000000000000000, 0.000000000000000000 ) ) ;
#2210=CARTESIAN_POINT ( 'NONE',  ( -73.06250000204840944, 80.81189881250001861, 10.69163855873948599 ) ) ;
#2218=CARTESIAN_POINT ( 'NONE',  ( -78.21875000204839523, 36.74823131438024859, -18.25176868561973720 ) ) ;
#2219=FACE_OUTER_BOUND ( 'NONE', #1580, .T. ) ;
#2224=CARTESIAN_POINT ( 'NONE',  ( -72.50000000409677625, 80.00000000000000000, -1.530808498934191324E-15 ) ) ;
#2226=DIRECTION ( 'NONE',  ( -1.000000000000000000, 0.000000000000000000, 0.000000000000000000 ) ) ;
#2231=ORIENTED_EDGE ( 'NONE', *, *, #4053, .T. ) ;
#2249=CYLINDRICAL_SURFACE ( 'NONE', #8030, 25.00000000000000355 ) ;
#2253=CARTESIAN_POINT ( 'NONE',  ( -79.71875000000001421, 80.00000000000001421, -10.35533905932737753 ) ) ;
#2256=FACE_OUTER_BOUND ( 'NONE', #11356, .T. ) ;
#2258=CARTESIAN_POINT ( 'NONE',  ( -75.00000000000000000, 55.00000000000000000, 0.000000000000000000 ) ) ;
#2270=CARTESIAN_POINT ( 'NONE',  ( -76.15625000000005684, 44.64466094067266511, 24.99999999999990408 ) ) ;
#2287=ORIENTED_EDGE ( 'NONE', *, *, #913, .T. ) ;
#2316=CARTESIAN_POINT ( 'NONE',  ( -71.99927368942448425, 76.65063862282433149, 12.49999388895319363 ) ) ;
#2319=DIRECTION ( 'NONE',  ( 0.000000000000000000, 0.000000000000000000, 1.000000000000000000 ) ) ;
#2332=CARTESIAN_POINT ( 'NONE',  ( -75.87500000204839523, 80.81189881250001861, 10.69163855873948599 ) ) ;
#2357=CARTESIAN_POINT ( 'NONE',  ( -73.34375000204839523, 55.00000000000000000, -25.81189881249999729 ) ) ;
#2358=CARTESIAN_POINT ( 'NONE',  ( -75.40624999999991473, 65.35533905933888832, -24.99999999998830802 ) ) ;
#2361=CARTESIAN_POINT ( 'NONE',  ( -75.00000000000001421, 31.19324792593015871, 8.552347646381322832 ) ) ;
#2372=CARTESIAN_POINT ( 'NONE',  ( -78.21875000204839523, 36.74823131438024859, -18.25176868561973720 ) ) ;
#2377=VERTEX_POINT ( 'NONE', #9184 ) ;
#2383=CARTESIAN_POINT ( 'NONE',  ( -76.25000000204838102, 65.69163855873948421, -25.81189881250000440 ) ) ;
#2390=CARTESIAN_POINT ( 'NONE',  ( -77.65625000204838102, 80.81189881250000440, -1.580522963032174394E-15 ) ) ;
#2394=CARTESIAN_POINT ( 'NONE',  ( -75.21875000409677625, 65.35533905932737753, 24.99999999999999645 ) ) ;
#2405=CARTESIAN_POINT ( 'NONE',  ( -78.87500000409677625, 55.00000000000000000, -24.99999999999999645 ) ) ;
#2412=CARTESIAN_POINT ( 'NONE',  ( -77.18750000204839523, 65.69163855873949842, 25.81189881250000440 ) ) ;
#2434=CARTESIAN_POINT ( 'NONE',  ( -77.37500000204838102, 65.69163855873949842, 25.81189881250000440 ) ) ;
#2448=CARTESIAN_POINT ( 'NONE',  ( -75.50000000204840944, 44.30836144126053000, 25.81189881250000795 ) ) ;
#2456=CARTESIAN_POINT ( 'NONE',  ( -77.28125000204838102, 55.00000000000000000, 25.81189881249999729 ) ) ;
#2469=PLANE ( 'NONE',  #9776 ) ;
#2476=ORIENTED_EDGE ( 'NONE', *, *, #2126, .T. ) ;
#2477=CARTESIAN_POINT ( 'NONE',  ( -75.96875000204839523, 80.81189881250000440, -1.580522963032174394E-15 ) ) ;
#2479=UNCERTAINTY_MEASURE_WITH_UNIT (LENGTH_MEASURE( 1.000000000000000082E-05 ), #11367, 'distance_accuracy_value', 'NONE');
#2486=CARTESIAN_POINT ( 'NONE',  ( -75.00000000000000000, 29.76427645923893550, -3.754450393707159161 ) ) ;
#2490=ORIENTED_EDGE ( 'NONE', *, *, #5858, .F. ) ;
#2497=CARTESIAN_POINT ( 'NONE',  ( -78.40625000204838102, 29.18810118750000271, 4.741568889096522788E-15 ) ) ;
#2502=DIRECTION ( 'NONE',  ( -1.000000000000000000, 0.000000000000000000, 0.000000000000000000 ) ) ;
#2512=CARTESIAN_POINT ( 'NONE',  ( -71.40810441781462714, 80.81189881250000440, 6.916273779317701376 ) ) ;
#2538=CARTESIAN_POINT ( 'NONE',  ( -76.81250000204839523, 29.18810118750000981, 10.69163855873950020 ) ) ;
#2543=CARTESIAN_POINT ( 'NONE',  ( -75.00000000000000000, 30.11944236376617567, -5.798191608586254375 ) ) ;
#2547=ORIENTED_EDGE ( 'NONE', *, *, #438, .F. ) ;
#2550=DIRECTION ( 'NONE',  ( -1.000000000000000000, 0.000000000000000000, 0.000000000000000000 ) ) ;
#2553=SURFACE_STYLE_FILL_AREA ( #3389 ) ;
#2560=EDGE_LOOP ( 'NONE', ( #601, #10241, #3736, #906 ) ) ;
#2564=DIRECTION ( 'NONE',  ( -1.000000000000000000, 0.000000000000000000, 0.000000000000000000 ) ) ;
#2579=CARTESIAN_POINT ( 'NONE',  ( -80.00000000000000000, 55.00000000000000000, -24.99999999999999645 ) ) ;
#2585=ORIENTED_EDGE ( 'NONE', *, *, #3159, .T. ) ;
#2596=CARTESIAN_POINT ( 'NONE',  ( -76.53125000204839523, 36.74823131438024859, -18.25176868561973720 ) ) ;
#2611=CARTESIAN_POINT ( 'NONE',  ( -74.93750000204839523, 65.69163855873948421, -25.81189881250000440 ) ) ;
#2623=DIRECTION ( 'NONE',  ( 0.000000000000000000, 0.000000000000000000, 1.000000000000000000 ) ) ;
#2636=DIRECTION ( 'NONE',  ( 0.000000000000000000, 0.000000000000000000, 1.000000000000000000 ) ) ;
#2639=CARTESIAN_POINT ( 'NONE',  ( -77.65625000204838102, 80.81189881250000440, -1.580522963032174394E-15 ) ) ;
#2647=CARTESIAN_POINT ( 'NONE',  ( -77.18750000204839523, 65.69163855873949842, 25.81189881250000084 ) ) ;
#2650=FACE_OUTER_BOUND ( 'NONE', #2560, .T. ) ;
#2654=CARTESIAN_POINT ( 'NONE',  ( -76.06250000409679046, 37.32233047033631124, -17.67766952966368166 ) ) ;
#2658=CARTESIAN_POINT ( 'NONE',  ( -77.18750000409679046, 72.67766952966368876, -17.67766952966368876 ) ) ;
#2672=CARTESIAN_POINT ( 'NONE',  ( -76.62500000000005684, 79.99999999999991473, -1.530808498934185605E-15 ) ) ;
#2676=ORIENTED_EDGE ( 'NONE', *, *, #8410, .T. ) ;
#2687=CARTESIAN_POINT ( 'NONE',  ( -83.00000000000000000, 55.00000000000000000, 0.000000000000000000 ) ) ;
#2702=CARTESIAN_POINT ( 'NONE',  ( -77.37500000204838102, 65.69163855873949842, 25.81189881250000440 ) ) ;
#2711=CARTESIAN_POINT ( 'NONE',  ( -75.21875000204839523, 29.18810118750000271, 4.741568889096522788E-15 ) ) ;
#2715=ORIENTED_EDGE ( 'NONE', *, *, #4119, .F. ) ;
#2717=CARTESIAN_POINT ( 'NONE',  ( -77.93750000409679046, 37.32233047033631124, 17.67766952966369232 ) ) ;
#2735=CARTESIAN_POINT ( 'NONE',  ( -76.90625000000005684, 65.35533905932732068, -24.99999999999990052 ) ) ;
#2758=CARTESIAN_POINT ( 'NONE',  ( -76.25000000204838102, 80.81189881250001861, -10.69163855873949132 ) ) ;
#2761=ORIENTED_EDGE ( 'NONE', *, *, #4332, .T. ) ;
#2764=CARTESIAN_POINT ( 'NONE',  ( -75.68750000204839523, 65.69163855873949842, 25.81189881250000084 ) ) ;
#2770=CARTESIAN_POINT ( 'NONE',  ( -77.65625000409677625, 30.00000000000000355, -10.35533905932738108 ) ) ;
#2785=CARTESIAN_POINT ( 'NONE',  ( -73.06250000204840944, 80.81189881250001861, 10.69163855873948599 ) ) ;
#2812=CARTESIAN_POINT ( 'NONE',  ( -75.50000000204840944, 29.18810118750000981, 10.69163855873950020 ) ) ;
#2820=DIRECTION ( 'NONE',  ( -1.000000000000000000, 0.000000000000000000, 0.000000000000000000 ) ) ;
#2824=ORIENTED_EDGE ( 'NONE', *, *, #7989, .F. ) ;
#2826=CARTESIAN_POINT ( 'NONE',  ( -71.75000000204840944, 65.69163855873948421, -25.81189881250000440 ) ) ;
#2846=ORIENTED_EDGE ( 'NONE', *, *, #307, .T. ) ;
#2858=VERTEX_POINT ( 'NONE', #694 ) ;
#2868=ORIENTED_EDGE ( 'NONE', *, *, #3159, .F. ) ;
#2876=CARTESIAN_POINT ( 'NONE',  ( -77.84375000204839523, 73.25176868561975141, -18.25176868561974430 ) ) ;
#2884=CARTESIAN_POINT ( 'NONE',  ( -75.50000000204840944, 44.30836144126052289, 25.81189881250000795 ) ) ;
#2885=CARTESIAN_POINT ( 'NONE',  ( -75.00000000000000000, 65.40507752864375846, -23.51498319519345159 ) ) ;
#2891=CARTESIAN_POINT ( 'NONE',  ( -77.46875000409679046, 44.64466094067260826, -24.99999999999998934 ) ) ;
#2902=ORIENTED_EDGE ( 'NONE', *, *, #8266, .T. ) ;
#2912=VERTEX_POINT ( 'NONE', #5090 ) ;
#2915=CARTESIAN_POINT ( 'NONE',  ( -79.53125000204838102, 55.00000000000000000, -25.81189881249999729 ) ) ;
#2924=CARTESIAN_POINT ( 'NONE',  ( -76.15624999999998579, 44.64466094067262958, 25.00000000000001066 ) ) ;
#2936=CARTESIAN_POINT ( 'NONE',  ( -73.90625000204838102, 29.18810118750000271, 4.741568889096522788E-15 ) ) ;
#2940=ADVANCED_FACE ( 'NONE', ( #3398 ), #6054, .F. ) ;
#2945=CARTESIAN_POINT ( 'NONE',  ( -75.00000000000001421, 58.46699551781524917, -25.57799957749213604 ) ) ;
#2981=CARTESIAN_POINT ( 'NONE',  ( -75.31250000000000000, 72.67766952966368876, -17.67766952966368876 ) ) ;
#2982=CARTESIAN_POINT ( 'NONE',  ( -75.00000000000000000, 54.23434559064500604, -25.81430454511032835 ) ) ;
#2994=CARTESIAN_POINT ( 'NONE',  ( -78.87500000204838102, 80.81189881250001861, 10.69163855873948599 ) ) ;
#3016=ORIENTED_EDGE ( 'NONE', *, *, #5885, .T. ) ;
#3036=CARTESIAN_POINT ( 'NONE',  ( -77.56250000409679046, 37.32233047033631124, -17.67766952966368166 ) ) ;
#3038=CARTESIAN_POINT ( 'NONE',  ( -75.49999999999972999, 55.00000000002793854, -24.99999999999999645 ) ) ;
#3041=CARTESIAN_POINT ( 'NONE',  ( -77.75000000000000000, 55.00000000000000000, 24.99999999999999645 ) ) ;
#3054=CARTESIAN_POINT ( 'NONE',  ( -78.12500000204838102, 29.18810118750000626, -10.69163855873949309 ) ) ;
#3058=CARTESIAN_POINT ( 'NONE',  ( -75.78125000000005684, 30.00000000000011013, -10.35533905932734022 ) ) ;
#3063=DIRECTION ( 'NONE',  ( 0.000000000000000000, 0.000000000000000000, 1.000000000000000000 ) ) ;
#3069=CARTESIAN_POINT ( 'NONE',  ( -72.68750000409677625, 72.67766952966368876, -17.67766952966368876 ) ) ;
#3094=( BOUNDED_CURVE ( )  B_SPLINE_CURVE ( 2, ( #2405, #6257, #6198, #4144, #544, #4208, #6020, #10660, #487 ),
 .UNSPECIFIED., .F., .T. ) 
 B_SPLINE_CURVE_WITH_KNOTS ( ( 3, 2, 2, 2, 3 ),
 ( 0.000000000000000000, 0.02083333333333334952, 0.04166666666666669905, 0.06250000000000005551, 0.08333333333333339810 ),
 .UNSPECIFIED. ) 
 CURVE ( )  GEOMETRIC_REPRESENTATION_ITEM ( )  RATIONAL_B_SPLINE_CURVE ( ( 1.000000000000000000, 0.9238795325112867385, 1.000000000000000000, 0.9238795325112867385, 1.000000000000000000, 0.9238795325112867385, 1.000000000000000000, 0.9238795325112865164, 1.000000000000000222 ) ) 
 REPRESENTATION_ITEM ( '' )  );
#3106=CARTESIAN_POINT ( 'NONE',  ( -77.00000000000000000, 55.00000000000000000, -24.99999999999999645 ) ) ;
#3114=DIRECTION ( 'NONE',  ( -1.000000000000000000, 0.000000000000000000, 0.000000000000000000 ) ) ;
#3117=CARTESIAN_POINT ( 'NONE',  ( -74.28125000204838102, 55.00000000000000000, 25.81189881249999729 ) ) ;
#3123=CARTESIAN_POINT ( 'NONE',  ( -78.40625000204838102, 29.18810118750000271, 4.741568889096522788E-15 ) ) ;
#3124=CARTESIAN_POINT ( 'NONE',  ( -75.00000000000001421, 77.22263599570800352, 11.53795789873604427 ) ) ;
#3126=ORIENTED_EDGE ( 'NONE', *, *, #9968, .F. ) ;
#3128=CARTESIAN_POINT ( 'NONE',  ( -73.43750000409677625, 37.32233047033631124, 17.67766952966369232 ) ) ;
#3130=ORIENTED_EDGE ( 'NONE', *, *, #799, .T. ) ;
#3148=PRODUCT_DEFINITION ( 'UNKNOWN', '', #6047, #11555 ) ;
#3154=CARTESIAN_POINT ( 'NONE',  ( -77.46875000409679046, 44.64466094067266511, -25.00000000000004263 ) ) ;
#3157=CARTESIAN_POINT ( 'NONE',  ( -78.12500000000000000, 80.00000000000000000, -1.530808498934191324E-15 ) ) ;
#3159=EDGE_CURVE ( 'NONE', #2858, #131, #1340, .T. ) ;
#3172=CARTESIAN_POINT ( 'NONE',  ( -77.46875000204839523, 80.81189881250000440, -1.580522963032174394E-15 ) ) ;
#3178=CARTESIAN_POINT ( 'NONE',  ( -75.00000000000001421, 58.46699551781524917, -25.57799957749213604 ) ) ;
#3184=CARTESIAN_POINT ( 'NONE',  ( -73.62500000409677625, 55.00000000000000000, 24.99999999999999645 ) ) ;
#3215=CARTESIAN_POINT ( 'NONE',  ( -77.56250000204838102, 80.81189881250001861, 10.69163855873948599 ) ) ;
#3216=CARTESIAN_POINT ( 'NONE',  ( -74.99999999999998579, 46.81069822181994056, -24.49304663887657796 ) ) ;
#3225=CARTESIAN_POINT ( 'NONE',  ( -75.00000000000000000, 55.00000000000000000, 25.00000000000000355 ) ) ;
#3228=CARTESIAN_POINT ( 'NONE',  ( -74.84375000204839523, 55.00000000000000000, -25.81189881249999729 ) ) ;
#3236=CARTESIAN_POINT ( 'NONE',  ( -75.00000000000000000, 76.68791387293471473, 12.43520775219157315 ) ) ;
#3248=CARTESIAN_POINT ( 'NONE',  ( -75.00000000000000000, 55.00000000000000000, 0.000000000000000000 ) ) ;
#3260=CARTESIAN_POINT ( 'NONE',  ( -75.00000000000001421, 42.56479188213557308, 21.68791366326873060 ) ) ;
#3272=CARTESIAN_POINT ( 'NONE',  ( -79.25000000204838102, 80.81189881250001861, -10.69163855873949132 ) ) ;
#3288=CARTESIAN_POINT ( 'NONE',  ( -76.15625000204839523, 73.25176868561975141, -18.25176868561974430 ) ) ;
#3292=AXIS2_PLACEMENT_3D ( 'NONE', #8167, #11808, #3434 ) ;
#3295=CARTESIAN_POINT ( 'NONE',  ( -75.21875000204839523, 36.74823131438024859, -18.25176868561973720 ) ) ;
#3316=CARTESIAN_POINT ( 'NONE',  ( -78.78125000204839523, 73.25176868561975141, 18.25176868561974075 ) ) ;
#3319=CARTESIAN_POINT ( 'NONE',  ( -75.00000000000000000, 55.00000000000000711, -29.00000000000000355 ) ) ;
#3325=ORIENTED_EDGE ( 'NONE', *, *, #4193, .T. ) ;
#3328=LINE ( 'NONE', #6277, #748 ) ;
#3330=CARTESIAN_POINT ( 'NONE',  ( -74.28125000000000000, 30.00000000000000355, -10.35533905932738108 ) ) ;
#3341=CARTESIAN_POINT ( 'NONE',  ( -72.03125000204839523, 36.74823131438024859, -18.25176868561973720 ) ) ;
#3348=CARTESIAN_POINT ( 'NONE',  ( -76.90625000204838102, 29.18810118750000271, 4.741568889096522788E-15 ) ) ;
#3354=EDGE_CURVE ( 'NONE', #8389, #5247, #11635, .T. ) ;
#3369=CARTESIAN_POINT ( 'NONE',  ( -77.37500000204838102, 80.81189881250001861, 10.69163855873948599 ) ) ;
#3387=CARTESIAN_POINT ( 'NONE',  ( -79.43750000204838102, 65.69163855873948421, -25.81189881250000440 ) ) ;
#3389=FILL_AREA_STYLE ('',( #5882 ) ) ;
#3395=( GEOMETRIC_REPRESENTATION_CONTEXT ( 3 ) GLOBAL_UNCERTAINTY_ASSIGNED_CONTEXT ( ( #5242 ) ) GLOBAL_UNIT_ASSIGNED_CONTEXT ( ( #6220, #5258, #5946 ) ) REPRESENTATION_CONTEXT ( 'NONE', 'WORKASPACE' ) );
#3398=FACE_OUTER_BOUND ( 'NONE', #3409, .T. ) ;
#3401=CARTESIAN_POINT ( 'NONE',  ( -75.00000000000000000, 55.00000000000000000, 0.000000000000000000 ) ) ;
#3402=CARTESIAN_POINT ( 'NONE',  ( -71.65625000204839523, 73.25176868561975141, -18.25176868561974430 ) ) ;
#3409=EDGE_LOOP ( 'NONE', ( #10070, #7159, #7399, #383 ) ) ;
#3410=CARTESIAN_POINT ( 'NONE',  ( -76.43750000204838102, 65.69163855873948421, -25.81189881250000084 ) ) ;
#3430=CARTESIAN_POINT ( 'NONE',  ( -74.46875000204839523, 80.81189881250000440, -1.580522963032174394E-15 ) ) ;
#3434=DIRECTION ( 'NONE',  ( 0.000000000000000000, 0.000000000000000000, 1.000000000000000000 ) ) ;
#3436=AXIS2_PLACEMENT_3D ( 'NONE', #3879, #8672, #2136 ) ;
#3439=CARTESIAN_POINT ( 'NONE',  ( -75.00000000000001421, 30.35902998560163013, -6.810003371955200890 ) ) ;
#3440=ORIENTED_EDGE ( 'NONE', *, *, #1274, .T. ) ;
#3448=CIRCLE ( 'NONE', #1908, 20.00000000000000355 ) ;
#3452=CARTESIAN_POINT ( 'NONE',  ( -77.65625000204838102, 80.81189881250000440, -1.580522963032174394E-15 ) ) ;
#3469=CARTESIAN_POINT ( 'NONE',  ( -72.68750000204839523, 65.69163855873949842, 25.81189881250000440 ) ) ;
#3487=EDGE_LOOP ( 'NONE', ( #2585, #7639, #1360, #3325 ) ) ;
#3490=DIRECTION ( 'NONE',  ( -1.000000000000000000, 0.000000000000000000, 0.000000000000000000 ) ) ;
#3495=CARTESIAN_POINT ( 'NONE',  ( -74.18750000204839523, 65.69163855873949842, 25.81189881250000440 ) ) ;
#3497=CARTESIAN_POINT ( 'NONE',  ( -76.71875000409676204, 65.35533905932729226, 25.00000000000008527 ) ) ;
#3500=CARTESIAN_POINT ( 'NONE',  ( -75.00000000000000000, 36.04064405738017740, 16.53539858576419519 ) ) ;
#3507=EDGE_LOOP ( 'NONE', ( #6227, #10207 ) ) ;
#3508=CARTESIAN_POINT ( 'NONE',  ( -77.00000000000000000, 55.00000000000000000, -24.99999999999999645 ) ) ;
#3518=CARTESIAN_POINT ( 'NONE',  ( -76.62500000409677625, 55.00000000000000000, 24.99999999999999645 ) ) ;
#3529=CARTESIAN_POINT ( 'NONE',  ( -75.00000000000000000, 55.00000000000000000, 25.00000000000000355 ) ) ;
#3535=CARTESIAN_POINT ( 'NONE',  ( -77.56250000204838102, 80.81189881250001861, 10.69163855873948599 ) ) ;
#3541=CARTESIAN_POINT ( 'NONE',  ( -78.12500000204839523, 29.18810118750000626, -10.69163855873949132 ) ) ;
#3542=( BOUNDED_CURVE ( )  B_SPLINE_CURVE ( 2, ( #5680, #2071, #9378, #7539, #11288, #2008, #3036, #3154, #4896 ),
 .UNSPECIFIED., .F., .T. ) 
 B_SPLINE_CURVE_WITH_KNOTS ( ( 3, 2, 2, 2, 3 ),
 ( 0.08333333333333339810, 0.1041666666666667546, 0.1250000000000001110, 0.1458333333333334814, 0.1666666666666667962 ),
 .UNSPECIFIED. ) 
 CURVE ( )  GEOMETRIC_REPRESENTATION_ITEM ( )  RATIONAL_B_SPLINE_CURVE ( ( 0.9999999999999997780, 0.9238795325112869605, 1.000000000000000000, 0.9238795325112867385, 1.000000000000000000, 0.9238795325112867385, 1.000000000000000000, 0.9238795325112861834, 1.000000000000000444 ) ) 
 REPRESENTATION_ITEM ( '' )  );
#3550=CARTESIAN_POINT ( 'NONE',  ( -78.68750000409679046, 72.67766952966368876, -17.67766952966368876 ) ) ;
#3568=CARTESIAN_POINT ( 'NONE',  ( -76.81250000000007105, 72.67766952966361771, -17.67766952966362126 ) ) ;
#3598=AXIS2_PLACEMENT_3D ( 'NONE', #7146, #11670, #2636 ) ;
#3604=CARTESIAN_POINT ( 'NONE',  ( -75.12500000204838102, 29.18810118750000626, -10.69163855873949132 ) ) ;
#3609=CARTESIAN_POINT ( 'NONE',  ( -76.53125000409679046, 44.64466094067255142, 24.99999999999992184 ) ) ;
#3610=CARTESIAN_POINT ( 'NONE',  ( -78.59375000409679046, 80.00000000000001421, -10.35533905932737753 ) ) ;
#3626=CARTESIAN_POINT ( 'NONE',  ( -72.87500000204839523, 65.69163855873949842, 25.81189881250000440 ) ) ;
#3638=DIRECTION ( 'NONE',  ( 0.000000000000000000, 0.000000000000000000, 1.000000000000000000 ) ) ;
#3664=CARTESIAN_POINT ( 'NONE',  ( -77.56250000204839523, 80.81189881250000440, -10.69163855873948954 ) ) ;
#3670=CARTESIAN_POINT ( 'NONE',  ( -75.12500000409677625, 55.00000000000000000, 24.99999999999999645 ) ) ;
#3685=CARTESIAN_POINT ( 'NONE',  ( -74.84375000204839523, 73.25176868561975141, -18.25176868561974430 ) ) ;
#3710=CARTESIAN_POINT ( 'NONE',  ( -75.59375000204839523, 36.74823131438026280, 18.25176868561974786 ) ) ;
#3717=CARTESIAN_POINT ( 'NONE',  ( -78.03125000204839523, 36.74823131438024859, -18.25176868561973720 ) ) ;
#3718=CARTESIAN_POINT ( 'NONE',  ( -75.00000000000000000, 66.33456766258404969, -23.06271704340218065 ) ) ;
#3723=CARTESIAN_POINT ( 'NONE',  ( -73.06250000204840944, 80.81189881250001861, -10.69163855873949132 ) ) ;
#3731=EDGE_CURVE ( 'NONE', #2912, #2858, #11488, .T. ) ;
#3736=ORIENTED_EDGE ( 'NONE', *, *, #4826, .T. ) ;
#3737=CARTESIAN_POINT ( 'NONE',  ( -75.78125000204838102, 55.00000000000000000, 25.81189881249999729 ) ) ;
#3756=DIRECTION ( 'NONE',  ( 0.000000000000000000, 0.000000000000000000, 1.000000000000000000 ) ) ;
#3764=ORIENTED_EDGE ( 'NONE', *, *, #9433, .F. ) ;
#3770=CARTESIAN_POINT ( 'NONE',  ( -75.40625000204838102, 29.18810118750000271, 4.741568889096522788E-15 ) ) ;
#3778=CARTESIAN_POINT ( 'NONE',  ( -79.25000000204839523, 65.69163855873948421, -25.81189881250000084 ) ) ;
#3779=CARTESIAN_POINT ( 'NONE',  ( -75.00000000000000000, 73.68484416130073100, -17.40076935087584076 ) ) ;
#3784=CARTESIAN_POINT ( 'NONE',  ( -78.31250000409679046, 72.67766952966368876, 17.67766952966368521 ) ) ;
#3792=EDGE_LOOP ( 'NONE', ( #10616, #3016, #10718 ) ) ;
#3793=CARTESIAN_POINT ( 'NONE',  ( -79.25000000000000000, 55.00000000000000000, 24.99999999999999645 ) ) ;
#3799=CARTESIAN_POINT ( 'NONE',  ( -76.53125000000004263, 79.99999999999990052, 10.35533905932733312 ) ) ;
#3819=CARTESIAN_POINT ( 'NONE',  ( -80.00000000000000000, 55.00000000000000000, -24.99999999999999645 ) ) ;
#3824=CIRCLE ( 'NONE', #936, 29.00000000000000355 ) ;
#3837=CARTESIAN_POINT ( 'NONE',  ( -74.09375000204839523, 36.74823131438026280, 18.25176868561974786 ) ) ;
#3864=( BOUNDED_SURFACE ( )  B_SPLINE_SURFACE ( 1, 2, ( 
 ( #3819, #4719, #6772, #2253, #1115, #275, #8373, #6590, #5866, #9505, #1233, #11350, #8496, #7488, #4963, #6712, #6825, #3882, #219, #1178, #3157, #10452, #11110, #9262, #3041, #9384, #11165, #7660, #397, #4902, #11293, #4845, #3106, #10220, #3938, #4000, #1297, #4779, #8618, #4065, #11231, #2924, #2012, #335, #9325, #10397, #8554, #7722, #8433, #7601, #2981, #6647, #2075, #5749, #10341, #2140, #5810, #5083, #8849, #9568, #7772, #3330, #510, #9682, #1361, #627, #4291, #5028, #8787, #9795, #11584, #8674, #568, #6999, #4173, #5991, #11643, #456, #8903, #9625, #9734, #7833, #1420, #7949, #4113, #11464, #2316, #685, #10571 ),
 ( #10622, #3387, #11402, #3272, #4358, #7062, #1532, #10512, #10686, #8728, #7894, #6103, #2497, #6945, #2372, #6045, #11524, #8009, #5256, #1477, #3452, #3215, #7122, #2434, #5138, #4236, #6162, #10745, #5198, #1588, #5925, #6883, #11708, #5428, #9133, #10973, #9911, #6447, #5546, #4527, #3737, #8295, #5484, #5313, #8239, #1814, #6392, #16, #855, #2611, #3685, #10021, #9189, #7175, #6337, #8183, #1707, #914, #6218, #4415, #11819, #9024, #9969, #9852, #4584, #7350, #1643, #9077, #10078, #2785, #8967, #3626, #7292, #801, #6280, #76, #742, #981, #5371, #1875, #4472, #8124, #4643, #8072, #11761, #10801, #7404, #7239, #10924 ) ),
 .UNSPECIFIED., .F., .F., .T. ) 
 B_SPLINE_SURFACE_WITH_KNOTS ( ( 2, 2 ),
 ( 3, 2, 2, 2, 2, 2, 2, 2, 2, 2, 2, 2, 2, 2, 2, 2, 2, 2, 2, 2, 2, 2, 2, 2, 2, 2, 2, 2, 2, 2, 2, 2, 2, 2, 2, 2, 2, 2, 2, 2, 2, 2, 2, 2, 3 ),
 ( 0.000000000000000000, 1.000000000000000000 ),
 ( 0.000000000000000000, 0.02083333333333333218, 0.04166666666666666435, 0.06250000000000000000, 0.08333333333333332871, 0.1041666666666666713, 0.1250000000000000000, 0.1458333333333333426, 0.1666666666666666574, 0.1875000000000000000, 0.2083333333333333426, 0.2291666666666666574, 0.2500000000000000000, 0.2708333333333333148, 0.2916666666666666852, 0.3125000000000000000, 0.3333333333333333148, 0.3541666666666666852, 0.3750000000000000000, 0.3958333333333333148, 0.4166666666666666852, 0.4375000000000000000, 0.4583333333333333148, 0.4791666666666666852, 0.5000000000000000000, 0.5208333333333333703, 0.5416666666666666297, 0.5625000000000000000, 0.5833333333333333703, 0.6041666666666666297, 0.6250000000000000000, 0.6458333333333333703, 0.6666666666666666297, 0.6875000000000000000, 0.7083333333333333703, 0.7291666666666666297, 0.7500000000000000000, 0.7708333333333333703, 0.7916666666666666297, 0.8125000000000000000, 0.8333333333333333703, 0.8541666666666666297, 0.8750000000000000000, 0.8888490471511721891, 0.8977375376226839343 ),
 .UNSPECIFIED. ) 
 GEOMETRIC_REPRESENTATION_ITEM ( )  RATIONAL_B_SPLINE_SURFACE ( (
 ( 1.000000000000000000, 0.9238795325112867385, 1.000000000000000000, 0.9238795325112867385, 1.000000000000000000, 0.9238795325112867385, 1.000000000000000000, 0.9238795325112867385, 1.000000000000000000, 0.9238795325112867385, 1.000000000000000000, 0.9238795325112867385, 1.000000000000000000, 0.9238795325112867385, 1.000000000000000000, 0.9238795325112867385, 1.000000000000000000, 0.9238795325112867385, 1.000000000000000000, 0.9238795325112867385, 1.000000000000000000, 0.9238795325112867385, 1.000000000000000000, 0.9238795325112867385, 1.000000000000000000, 0.9238795325112867385, 1.000000000000000000, 0.9238795325112867385, 1.000000000000000000, 0.9238795325112867385, 1.000000000000000000, 0.9238795325112867385, 1.000000000000000000, 0.9238795325112867385, 1.000000000000000000, 0.9238795325112867385, 1.000000000000000000, 0.9238795325112867385, 1.000000000000000000, 0.9238795325112867385, 1.000000000000000000, 0.9238795325112867385, 1.000000000000000000, 0.9238795325112867385, 1.000000000000000000, 0.9238795325112867385, 1.000000000000000000, 0.9238795325112867385, 1.000000000000000000, 0.9238795325112867385, 1.000000000000000000, 0.9238795325112867385, 1.000000000000000000, 0.9238795325112867385, 1.000000000000000000, 0.9238795325112867385, 1.000000000000000000, 0.9238795325112867385, 1.000000000000000000, 0.9238795325112867385, 1.000000000000000000, 0.9238795325112867385, 1.000000000000000000, 0.9238795325112867385, 1.000000000000000000, 0.9238795325112867385, 1.000000000000000000, 0.9238795325112867385, 1.000000000000000000, 0.9238795325112867385, 1.000000000000000000, 0.9238795325112867385, 1.000000000000000000, 0.9238795325112867385, 1.000000000000000000, 0.9238795325112867385, 1.000000000000000000, 0.9238795325112867385, 1.000000000000000000, 0.9238795325112867385, 1.000000000000000000, 0.9238795325112867385, 1.000000000000000000, 0.9238795325112867385, 1.000000000000000000, 0.9493985947158180005, 0.9660721892104719988, 0.9660721892104719988, 0.9660721892104719988),
 ( 1.000000000000000000, 0.9238795325112867385, 1.000000000000000000, 0.9238795325112867385, 1.000000000000000000, 0.9238795325112867385, 1.000000000000000000, 0.9238795325112867385, 1.000000000000000000, 0.9238795325112867385, 1.000000000000000000, 0.9238795325112867385, 1.000000000000000000, 0.9238795325112867385, 1.000000000000000000, 0.9238795325112867385, 1.000000000000000000, 0.9238795325112867385, 1.000000000000000000, 0.9238795325112867385, 1.000000000000000000, 0.9238795325112867385, 1.000000000000000000, 0.9238795325112867385, 1.000000000000000000, 0.9238795325112867385, 1.000000000000000000, 0.9238795325112867385, 1.000000000000000000, 0.9238795325112867385, 1.000000000000000000, 0.9238795325112867385, 1.000000000000000000, 0.9238795325112867385, 1.000000000000000000, 0.9238795325112867385, 1.000000000000000000, 0.9238795325112867385, 1.000000000000000000, 0.9238795325112867385, 1.000000000000000000, 0.9238795325112867385, 1.000000000000000000, 0.9238795325112867385, 1.000000000000000000, 0.9238795325112867385, 1.000000000000000000, 0.9238795325112867385, 1.000000000000000000, 0.9238795325112867385, 1.000000000000000000, 0.9238795325112867385, 1.000000000000000000, 0.9238795325112867385, 1.000000000000000000, 0.9238795325112867385, 1.000000000000000000, 0.9238795325112867385, 1.000000000000000000, 0.9238795325112867385, 1.000000000000000000, 0.9238795325112867385, 1.000000000000000000, 0.9238795325112867385, 1.000000000000000000, 0.9238795325112867385, 1.000000000000000000, 0.9238795325112867385, 1.000000000000000000, 0.9238795325112867385, 1.000000000000000000, 0.9238795325112867385, 1.000000000000000000, 0.9238795325112867385, 1.000000000000000000, 0.9238795325112867385, 1.000000000000000000, 0.9238795325112867385, 1.000000000000000000, 0.9238795325112867385, 1.000000000000000000, 0.9238795325112867385, 1.000000000000000000, 0.9238795325112867385, 1.000000000000000000, 0.9493985947158180005, 0.9660721892104719988, 0.9660721892104719988, 0.9660721892104719988) ) ) 
 REPRESENTATION_ITEM ( '' )  SURFACE ( )  );
#3879=CARTESIAN_POINT ( 'NONE',  ( -75.00000000000000000, 55.00000000000000000, 0.000000000000000000 ) ) ;
#3882=CARTESIAN_POINT ( 'NONE',  ( -78.40625000000000000, 65.35533905932737753, -24.99999999999999645 ) ) ;
#3895=CARTESIAN_POINT ( 'NONE',  ( -72.68750000204839523, 44.30836144126053000, 25.81189881250000795 ) ) ;
#3907=CARTESIAN_POINT ( 'NONE',  ( -73.25000000409677625, 30.00000000000000355, 4.592425496802573578E-15 ) ) ;
#3912=DIRECTION ( 'NONE',  ( -1.000000000000000000, 0.000000000000000000, 0.000000000000000000 ) ) ;
#3938=CARTESIAN_POINT ( 'NONE',  ( -76.81250000000000000, 72.67766952966368876, -17.67766952966368876 ) ) ;
#3952=CARTESIAN_POINT ( 'NONE',  ( -71.84375000204838102, 73.25176868561975141, -18.25176868561974430 ) ) ;
#3961=DIRECTION ( 'NONE',  ( -1.000000000000000000, 0.000000000000000000, 0.000000000000000000 ) ) ;
#3968=CARTESIAN_POINT ( 'NONE',  ( -72.31250000409677625, 72.67766952966368876, 17.67766952966368521 ) ) ;
#3994=CARTESIAN_POINT ( 'NONE',  ( -79.15625000000001421, 44.64466094067263668, 24.99999999999997513 ) ) ;
#4000=CARTESIAN_POINT ( 'NONE',  ( -76.71875000000000000, 80.00000000000001421, -10.35533905932737753 ) ) ;
#4012=EDGE_CURVE ( 'NONE', #5247, #1715, #3094, .T. ) ;
#4014=CARTESIAN_POINT ( 'NONE',  ( -74.46875000204839523, 73.25176868561975141, 18.25176868561974075 ) ) ;
#4028=CARTESIAN_POINT ( 'NONE',  ( -71.56250000409677625, 37.32233047033631124, -17.67766952966368166 ) ) ;
#4053=EDGE_CURVE ( 'NONE', #8475, #7495, #4314, .T. ) ;
#4065=CARTESIAN_POINT ( 'NONE',  ( -76.34375000000001421, 65.35533905932737753, 24.99999999999999645 ) ) ;
#4066=CARTESIAN_POINT ( 'NONE',  ( -74.99999999999998579, 39.36515909056227258, -20.53791299142420712 ) ) ;
#4075=CARTESIAN_POINT ( 'NONE',  ( -78.31250000204839523, 29.18810118750000981, 10.69163855873950020 ) ) ;
#4079=CARTESIAN_POINT ( 'NONE',  ( -79.25000000204839523, 80.81189881250000440, -10.69163855873948954 ) ) ;
#4084=CARTESIAN_POINT ( 'NONE',  ( -71.28125000409677625, 65.35533905932737753, -24.99999999999999645 ) ) ;
#4111=ADVANCED_FACE ( 'NONE', ( #5234, #6976 ), #2469, .T. ) ;
#4112=ORIENTED_EDGE ( 'NONE', *, *, #1668, .F. ) ;
#4113=CARTESIAN_POINT ( 'NONE',  ( -72.12500000000000000, 80.00000000000000000, -1.530808498934191324E-15 ) ) ;
#4114=CARTESIAN_POINT ( 'NONE',  ( -75.00000000000002842, 40.04116987730228772, -21.05253787605388638 ) ) ;
#4119=EDGE_CURVE ( 'NONE', #9864, #9375, #11484, .T. ) ;
#4121=DIRECTION ( 'NONE',  ( 0.000000000000000000, 0.000000000000000000, -1.000000000000000000 ) ) ;
#4125=CARTESIAN_POINT ( 'NONE',  ( -74.28125000204839523, 73.25176868561975141, 18.25176868561974075 ) ) ;
#4134=CARTESIAN_POINT ( 'NONE',  ( -75.00000000000000000, 55.00000000000000000, 0.000000000000000000 ) ) ;
#4144=CARTESIAN_POINT ( 'NONE',  ( -78.59375000409677625, 80.00000000000001421, -10.35533905932737753 ) ) ;
#4161=CARTESIAN_POINT ( 'NONE',  ( -75.06471690751966719, 48.34131301757658150, 24.99999999999992184 ) ) ;
#4173=CARTESIAN_POINT ( 'NONE',  ( -73.06250000000000000, 37.32233047033631124, 17.67766952966369232 ) ) ;
#4186=CARTESIAN_POINT ( 'NONE',  ( -73.71875000204839523, 29.18810118750000271, 4.741568889096522788E-15 ) ) ;
#4192=CARTESIAN_POINT ( 'NONE',  ( -75.59374999999990052, 44.64466094068421143, -25.00000000001146105 ) ) ;
#4193=EDGE_CURVE ( 'NONE', #8389, #2858, #5540, .T. ) ;
#4195=CARTESIAN_POINT ( 'NONE',  ( -75.50000000204840944, 29.18810118750000981, 10.69163855873950020 ) ) ;
#4208=CARTESIAN_POINT ( 'NONE',  ( -78.40625000409677625, 80.00000000000001421, 10.35533905932737397 ) ) ;
#4215=CARTESIAN_POINT ( 'NONE',  ( -77.75000000204839523, 65.69163855873948421, -25.81189881250000440 ) ) ;
#4221=CARTESIAN_POINT ( 'NONE',  ( -74.99999999999998579, 39.36515909056227258, -20.53791299142420712 ) ) ;
#4225=EDGE_CURVE ( 'NONE', #7521, #2004, #9169, .T. ) ;
#4233=AXIS2_PLACEMENT_3D ( 'NONE', #10424, #2226, #11436 ) ;
#4236=CARTESIAN_POINT ( 'NONE',  ( -77.18750000204838102, 44.30836144126053000, 25.81189881250000795 ) ) ;
#4249=CARTESIAN_POINT ( 'NONE',  ( -72.59375000204838102, 55.00000000000000000, 25.81189881249999729 ) ) ;
#4256=CARTESIAN_POINT ( 'NONE',  ( -77.09375000204839523, 36.74823131438026280, 18.25176868561974786 ) ) ;
#4270=CARTESIAN_POINT ( 'NONE',  ( -77.65624999999998579, 44.64466094066740709, 24.99999999999465672 ) ) ;
#4276=CARTESIAN_POINT ( 'NONE',  ( -75.78125000204839523, 73.25176868561975141, 18.25176868561974075 ) ) ;
#4291=CARTESIAN_POINT ( 'NONE',  ( -73.81250000000000000, 72.67766952966368876, -17.67766952966368876 ) ) ;
#4301=LINE ( 'NONE', #4427, #8118 ) ;
#4303=CARTESIAN_POINT ( 'NONE',  ( -74.75000000204840944, 65.69163855873948421, -25.81189881250000440 ) ) ;
#4311=CARTESIAN_POINT ( 'NONE',  ( -76.62500000204838102, 44.30836144126049447, -25.81189881249999019 ) ) ;
#4314=( BOUNDED_CURVE ( )  B_SPLINE_CURVE ( 2, ( #1450, #4270, #11502, #7807, #7870, #10601, #7983, #1509, #4327 ),
 .UNSPECIFIED., .F., .T. ) 
 B_SPLINE_CURVE_WITH_KNOTS ( ( 3, 2, 2, 2, 3 ),
 ( 0.2376281879409543607, 0.2574394709827818040, 0.2772507540246093027, 0.2970620370664368015, 0.3168733201082642448 ),
 .UNSPECIFIED. ) 
 CURVE ( )  GEOMETRIC_REPRESENTATION_ITEM ( )  RATIONAL_B_SPLINE_CURVE ( ( 0.9999999999999494849, 0.9238795325113373647, 1.000000000000000000, 0.9238795325112868495, 1.000000000000000000, 0.9238795325112868495, 1.000000000000000000, 0.9238795325112868495, 1.000000000000000000 ) ) 
 REPRESENTATION_ITEM ( '' )  );
#4320=CARTESIAN_POINT ( 'NONE',  ( -80.00000000000000000, 55.00000000000000000, 0.000000000000000000 ) ) ;
#4327=CARTESIAN_POINT ( 'NONE',  ( -77.00000000000000000, 55.00000000000000000, -24.99999999999999645 ) ) ;
#4332=EDGE_CURVE ( 'NONE', #9420, #8886, #5709, .T. ) ;
#4338=CARTESIAN_POINT ( 'NONE',  ( -74.65625000204839523, 73.25176868561975141, -18.25176868561974430 ) ) ;
#4341=ADVANCED_FACE ( 'NONE', ( #4985, #354 ), #8636, .F. ) ;
#4345=CARTESIAN_POINT ( 'NONE',  ( -75.00000000000000000, 32.46325592683887606, 11.40855839108016667 ) ) ;
#4358=CARTESIAN_POINT ( 'NONE',  ( -79.15625000204838102, 80.81189881250000440, -1.580522963032174394E-15 ) ) ;
#4363=MECHANICAL_DESIGN_GEOMETRIC_PRESENTATION_REPRESENTATION('',(#6669),#2050);
#4369=CARTESIAN_POINT ( 'NONE',  ( -72.31250000204839523, 29.18810118750000981, 10.69163855873950020 ) ) ;
#4377=CARTESIAN_POINT ( 'NONE',  ( -77.46875000204839523, 73.25176868561975141, 18.25176868561974075 ) ) ;
#4379=EDGE_CURVE ( 'NONE', #5071, #131, #9971, .T. ) ;
#4398=CARTESIAN_POINT ( 'NONE',  ( -74.28125000204839523, 73.25176868561975141, 18.25176868561974075 ) ) ;
#4406=CARTESIAN_POINT ( 'NONE',  ( -74.99999999999994316, 33.80523199205565277, 13.63254922431209870 ) ) ;
#4415=CARTESIAN_POINT ( 'NONE',  ( -74.00000000204839523, 29.18810118750000981, 10.69163855873950020 ) ) ;
#4427=CARTESIAN_POINT ( 'NONE',  ( -75.00000000000000000, 55.00000000000000000, 25.00000000000000355 ) ) ;
#4429=CARTESIAN_POINT ( 'NONE',  ( -83.00000000000000000, 55.00000000000000000, 0.000000000000000000 ) ) ;
#4446=CARTESIAN_POINT ( 'NONE',  ( -74.75000000204839523, 80.81189881250001861, -10.69163855873949132 ) ) ;
#4452=CARTESIAN_POINT ( 'NONE',  ( -79.06250000204840944, 80.81189881250000440, -10.69163855873948954 ) ) ;
#4454=CARTESIAN_POINT ( 'NONE',  ( -83.00000000000000000, 55.00000000000000000, 0.000000000000000000 ) ) ;
#4458=CARTESIAN_POINT ( 'NONE',  ( -77.93750000204838102, 44.30836144126050158, -25.81189881249999374 ) ) ;
#4461=CARTESIAN_POINT ( 'NONE',  ( -80.00000000000000000, 55.00000000000000000, 20.00000000000000355 ) ) ;
#4472=CARTESIAN_POINT ( 'NONE',  ( -72.03125000204838102, 55.00000000000000000, -25.81189881249999729 ) ) ;
#4477=ORIENTED_EDGE ( 'NONE', *, *, #6659, .F. ) ;
#4504=CARTESIAN_POINT ( 'NONE',  ( -75.96875000204839523, 80.81189881250000440, -1.580522963032174394E-15 ) ) ;
#4506=DIRECTION ( 'NONE',  ( 1.000000000000000000, -0.000000000000000000, -0.000000000000000000 ) ) ;
#4509=CARTESIAN_POINT ( 'NONE',  ( -77.09375000409677625, 80.00000000000001421, -10.35533905932737753 ) ) ;
#4527=CARTESIAN_POINT ( 'NONE',  ( -75.87500000204839523, 65.69163855873949842, 25.81189881250000440 ) ) ;
#4537=DIRECTION ( 'NONE',  ( -1.000000000000000000, -0.000000000000000000, -0.000000000000000000 ) ) ;
#4540=DIRECTION ( 'NONE',  ( 0.000000000000000000, 0.000000000000000000, 1.000000000000000000 ) ) ;
#4558=CARTESIAN_POINT ( 'NONE',  ( -77.09375000204839523, 36.74823131438026280, 18.25176868561974786 ) ) ;
#4559=CIRCLE ( 'NONE', #3598, 20.00000000000000355 ) ;
#4560=ORIENTED_EDGE ( 'NONE', *, *, #6659, .T. ) ;
#4567=CARTESIAN_POINT ( 'NONE',  ( -78.68750000204839523, 65.69163855873949842, 25.81189881250000084 ) ) ;
#4571=CARTESIAN_POINT ( 'NONE',  ( -78.87500000409677625, 55.00000000000000000, -24.99999999999999645 ) ) ;
#4579=EDGE_LOOP ( 'NONE', ( #9581, #6344, #2846, #4755 ) ) ;
#4583=VERTEX_POINT ( 'NONE', #7313 ) ;
#4584=CARTESIAN_POINT ( 'NONE',  ( -73.53125000204838102, 55.00000000000000000, -25.81189881249999729 ) ) ;
#4594=CYLINDRICAL_SURFACE ( 'NONE', #11352, 29.00000000000000355 ) ;
#4612=CARTESIAN_POINT ( 'NONE',  ( -77.46875000204839523, 73.25176868561975141, 18.25176868561974075 ) ) ;
#4620=CARTESIAN_POINT ( 'NONE',  ( -76.81250000204839523, 29.18810118750000981, 10.69163855873950020 ) ) ;
#4622=CYLINDRICAL_SURFACE ( 'NONE', #10076, 20.00000000000000355 ) ;
#4628=CARTESIAN_POINT ( 'NONE',  ( -78.03125000409677625, 44.64466094067262958, 25.00000000000001066 ) ) ;
#4643=CARTESIAN_POINT ( 'NONE',  ( -71.84375000204838102, 73.25176868561975141, -18.25176868561974430 ) ) ;
#4648=CYLINDRICAL_SURFACE ( 'NONE', #4805, 25.00000000000000355 ) ;
#4669=CARTESIAN_POINT ( 'NONE',  ( -75.03125000204838102, 55.00000000000000000, -25.81189881249999729 ) ) ;
#4677=CARTESIAN_POINT ( 'NONE',  ( -77.93750000204838102, 44.30836144126049447, -25.81189881249999019 ) ) ;
#4678=CARTESIAN_POINT ( 'NONE',  ( -75.00000000000000000, 80.04891742985661551, -3.510137850074999122 ) ) ;
#4682=CARTESIAN_POINT ( 'NONE',  ( -72.40625000204839523, 36.74823131438026280, 18.25176868561974786 ) ) ;
#4694=CARTESIAN_POINT ( 'NONE',  ( -75.00000000000000000, 55.00000000000000711, -29.00000000000000355 ) ) ;
#4715=AXIS2_PLACEMENT_3D ( 'NONE', #11085, #3912, #7578 ) ;
#4719=CARTESIAN_POINT ( 'NONE',  ( -79.90625000000000000, 65.35533905932737753, -24.99999999999999645 ) ) ;
#4733=CARTESIAN_POINT ( 'NONE',  ( -72.59375000204838102, 36.74823131438026280, 18.25176868561974786 ) ) ;
#4738=AXIS2_PLACEMENT_3D ( 'NONE', #6164, #8011, #1383 ) ;
#4743=CARTESIAN_POINT ( 'NONE',  ( -74.99999999999998579, 79.48388272459020243, -6.547252175383230899 ) ) ;
#4748=CARTESIAN_POINT ( 'NONE',  ( -76.34375000409680467, 30.00000000000001421, 10.35533905932739174 ) ) ;
#4755=ORIENTED_EDGE ( 'NONE', *, *, #4012, .F. ) ;
#4776=CARTESIAN_POINT ( 'NONE',  ( -75.21875000409676204, 65.35533905932724963, 25.00000000000012434 ) ) ;
#4779=CARTESIAN_POINT ( 'NONE',  ( -76.53124999999998579, 80.00000000000001421, 10.35533905932737397 ) ) ;
#4789=UNCERTAINTY_MEASURE_WITH_UNIT (LENGTH_MEASURE( 1.000000000000000082E-05 ), #10005, 'distance_accuracy_value', 'NONE');
#4795=CARTESIAN_POINT ( 'NONE',  ( -73.15625000204838102, 80.81189881250000440, -1.580522963032174394E-15 ) ) ;
#4802=CARTESIAN_POINT ( 'NONE',  ( -79.15625000204838102, 80.81189881250000440, -1.580522963032174394E-15 ) ) ;
#4804=CARTESIAN_POINT ( 'NONE',  ( -74.99999999999998579, 74.03124084216746326, -17.00900853765869059 ) ) ;
#4805=AXIS2_PLACEMENT_3D ( 'NONE', #2067, #8423, #2128 ) ;
#4811=DIRECTION ( 'NONE',  ( 0.000000000000000000, 0.000000000000000000, 1.000000000000000000 ) ) ;
#4826=EDGE_CURVE ( 'NONE', #11373, #10439, #400, .T. ) ;
#4843=ADVANCED_FACE ( 'NONE', ( #2256 ), #9798, .F. ) ;
#4845=CARTESIAN_POINT ( 'NONE',  ( -77.09374999999998579, 44.64466094067260826, -24.99999999999998934 ) ) ;
#4858=CARTESIAN_POINT ( 'NONE',  ( -77.84375000204839523, 55.00000000000000000, -25.81189881249999729 ) ) ;
#4870=CARTESIAN_POINT ( 'NONE',  ( -73.15625000409677625, 30.00000000000000355, -10.35533905932738108 ) ) ;
#4885=CARTESIAN_POINT ( 'NONE',  ( -79.34375000204839523, 55.00000000000000000, -25.81189881249999729 ) ) ;
#4896=CARTESIAN_POINT ( 'NONE',  ( -77.37500000409677625, 55.00000000000000000, -24.99999999999999645 ) ) ;
#4899=CARTESIAN_POINT ( 'NONE',  ( -75.78125000409680467, 65.35533905932749121, -24.99999999999989342 ) ) ;
#4902=CARTESIAN_POINT ( 'NONE',  ( -77.28124999999998579, 30.00000000000000355, -10.35533905932738108 ) ) ;
#4903=CARTESIAN_POINT ( 'NONE',  ( -74.99999999999997158, 50.05679712599850006, -25.38984111367952679 ) ) ;
#4916=CARTESIAN_POINT ( 'NONE',  ( -74.37500000204838102, 65.69163855873949842, 25.81189881250000440 ) ) ;
#4920=CARTESIAN_POINT ( 'NONE',  ( -76.25000000000000000, 55.00000000000000000, 24.99999999999999645 ) ) ;
#4930=CARTESIAN_POINT ( 'NONE',  ( -73.90625000409680467, 80.00000000000001421, 10.35533905932737397 ) ) ;
#4944=APPLICATION_CONTEXT ( 'automotive_design' ) ;
#4963=CARTESIAN_POINT ( 'NONE',  ( -78.68750000000001421, 37.32233047033631124, -17.67766952966368166 ) ) ;
#4977=CARTESIAN_POINT ( 'NONE',  ( -79.25000000204838102, 65.69163855873948421, -25.81189881250000440 ) ) ;
#4985=FACE_OUTER_BOUND ( 'NONE', #8973, .T. ) ;
#5025=CARTESIAN_POINT ( 'NONE',  ( -75.12500000409677625, 55.00000000000000000, 24.99999999999999645 ) ) ;
#5027=ORIENTED_EDGE ( 'NONE', *, *, #9234, .F. ) ;
#5028=CARTESIAN_POINT ( 'NONE',  ( -73.71875000000000000, 80.00000000000001421, -10.35533905932737753 ) ) ;
#5039=CARTESIAN_POINT ( 'NONE',  ( -75.59375000204839523, 55.00000000000000000, 25.81189881249999729 ) ) ;
#5044=SURFACE_STYLE_USAGE ( .BOTH. , #9525 ) ;
#5059=ORIENTED_EDGE ( 'NONE', *, *, #4379, .T. ) ;
#5071=VERTEX_POINT ( 'NONE', #11711 ) ;
#5083=CARTESIAN_POINT ( 'NONE',  ( -74.65625000000000000, 44.64466094067262958, 25.00000000000001066 ) ) ;
#5088=ORIENTED_EDGE ( 'NONE', *, *, #55, .F. ) ;
#5090=CARTESIAN_POINT ( 'NONE',  ( -75.00000000000001421, 42.56479188213557308, 21.68791366326873060 ) ) ;
#5095=CARTESIAN_POINT ( 'NONE',  ( -74.65625000204839523, 73.25176868561975141, -18.25176868561974430 ) ) ;
#5104=CARTESIAN_POINT ( 'NONE',  ( -75.49999999999972999, 55.00000000002793854, -24.99999999999999645 ) ) ;
#5112=EDGE_LOOP ( 'NONE', ( #2231, #7849, #675, #9188 ) ) ;
#5123=CARTESIAN_POINT ( 'NONE',  ( -73.81250000204839523, 29.18810118750000981, 10.69163855873950020 ) ) ;
#5129=CARTESIAN_POINT ( 'NONE',  ( -75.00000000000000000, 31.58343112012256526, 9.522673556080674118 ) ) ;
#5138=CARTESIAN_POINT ( 'NONE',  ( -77.28125000204838102, 55.00000000000000000, 25.81189881249999729 ) ) ;
#5151=CARTESIAN_POINT ( 'NONE',  ( -73.25000000204839523, 65.69163855873948421, -25.81189881250000440 ) ) ;
#5157=CARTESIAN_POINT ( 'NONE',  ( -75.40625000204838102, 29.18810118750000271, 4.741568889096522788E-15 ) ) ;
#5171=DIRECTION ( 'NONE',  ( -1.000000000000000000, 0.000000000000000000, 0.000000000000000000 ) ) ;
#5178=CARTESIAN_POINT ( 'NONE',  ( -78.12500000204838102, 29.18810118750000626, -10.69163855873949309 ) ) ;
#5196=VECTOR ( 'NONE', #2820, 1000.000000000000000 ) ;
#5198=CARTESIAN_POINT ( 'NONE',  ( -76.90625000204838102, 29.18810118750000271, 4.741568889096522788E-15 ) ) ;
#5208=DIRECTION ( 'NONE',  ( 1.000000000000000000, -0.000000000000000000, -0.000000000000000000 ) ) ;
#5212=CARTESIAN_POINT ( 'NONE',  ( -75.21875000204839523, 29.18810118750000271, 4.741568889096522788E-15 ) ) ;
#5221=CARTESIAN_POINT ( 'NONE',  ( -75.68750000204838102, 44.30836144126052289, 25.81189881250000795 ) ) ;
#5226=CARTESIAN_POINT ( 'NONE',  ( -77.75000000000000000, 55.00000000000000000, 24.99999999999999645 ) ) ;
#5228=DIRECTION ( 'NONE',  ( -1.000000000000000000, 0.000000000000000000, 0.000000000000000000 ) ) ;
#5229=ORIENTED_EDGE ( 'NONE', *, *, #10606, .F. ) ;
#5234=FACE_OUTER_BOUND ( 'NONE', #7001, .T. ) ;
#5240=CARTESIAN_POINT ( 'NONE',  ( -74.93750000204839523, 44.30836144126050158, -25.81189881249999374 ) ) ;
#5242=UNCERTAINTY_MEASURE_WITH_UNIT (LENGTH_MEASURE( 1.000000000000000082E-05 ), #6220, 'distance_accuracy_value', 'NONE');
#5246=CARTESIAN_POINT ( 'NONE',  ( -75.00000000000000000, 29.54384304976292697, -0.6381725101535358213 ) ) ;
#5247=VERTEX_POINT ( 'NONE', #8827 ) ;
#5256=CARTESIAN_POINT ( 'NONE',  ( -77.84375000204839523, 73.25176868561975141, -18.25176868561974430 ) ) ;
#5258=( NAMED_UNIT ( * ) PLANE_ANGLE_UNIT ( ) SI_UNIT ( $, .RADIAN. ) );
#5296=CARTESIAN_POINT ( 'NONE',  ( -75.40625000204839523, 36.74823131438026280, 18.25176868561974786 ) ) ;
#5307=ORIENTED_EDGE ( 'NONE', *, *, #4225, .F. ) ;
#5313=CARTESIAN_POINT ( 'NONE',  ( -75.50000000204840944, 29.18810118750000981, 10.69163855873950020 ) ) ;
#5315=( NAMED_UNIT ( * ) SI_UNIT ( $, .STERADIAN. ) SOLID_ANGLE_UNIT ( ) );
#5324=CARTESIAN_POINT ( 'NONE',  ( -83.00000000000000000, 55.00000000000000000, 0.000000000000000000 ) ) ;
#5342=CARTESIAN_POINT ( 'NONE',  ( -75.78125000204838102, 55.00000000000000000, 25.81189881249999729 ) ) ;
#5355=CARTESIAN_POINT ( 'NONE',  ( -75.50000000204840944, 44.30836144126053000, 25.81189881250000795 ) ) ;
#5371=CARTESIAN_POINT ( 'NONE',  ( -72.21875000204838102, 36.74823131438024859, -18.25176868561973720 ) ) ;
#5377=CARTESIAN_POINT ( 'NONE',  ( -75.00000000000000000, 55.00000000000000000, 0.000000000000000000 ) ) ;
#5384=CARTESIAN_POINT ( 'NONE',  ( -75.00000000000000000, 55.00000000000000000, 0.000000000000000000 ) ) ;
#5401=CARTESIAN_POINT ( 'NONE',  ( -77.75000000204839523, 80.81189881250001861, -10.69163855873949132 ) ) ;
#5404=VERTEX_POINT ( 'NONE', #6618 ) ;
#5407=CARTESIAN_POINT ( 'NONE',  ( -76.25000000204838102, 65.69163855873948421, -25.81189881250000084 ) ) ;
#5412=CARTESIAN_POINT ( 'NONE',  ( -76.15625000409677625, 30.00000000000000355, -10.35533905932738108 ) ) ;
#5413=CARTESIAN_POINT ( 'NONE',  ( -75.78125000409680467, 65.35533905932737753, -24.99999999999999645 ) ) ;
#5428=CARTESIAN_POINT ( 'NONE',  ( -76.43750000204838102, 65.69163855873948421, -25.81189881250000440 ) ) ;
#5462=CARTESIAN_POINT ( 'NONE',  ( -76.15625000204839523, 73.25176868561975141, -18.25176868561974430 ) ) ;
#5468=CARTESIAN_POINT ( 'NONE',  ( -77.56250000409679046, 37.32233047033631124, -17.67766952966368166 ) ) ;
#5484=CARTESIAN_POINT ( 'NONE',  ( -75.59375000204839523, 36.74823131438026280, 18.25176868561974786 ) ) ;
#5514=CARTESIAN_POINT ( 'NONE',  ( -79.15625000204838102, 80.81189881250000440, -1.580522963032174394E-15 ) ) ;
#5521=CARTESIAN_POINT ( 'NONE',  ( -75.87500000204838102, 80.81189881250000440, 10.69163855873948243 ) ) ;
#5523=DIRECTION ( 'NONE',  ( 0.000000000000000000, -1.000000000000000000, 0.000000000000000000 ) ) ;
#5526=CARTESIAN_POINT ( 'NONE',  ( -72.03125000204839523, 36.74823131438024859, -18.25176868561973720 ) ) ;
#5540=( BOUNDED_CURVE ( )  B_SPLINE_CURVE ( 2, ( #1854, #3778, #8328, #4452, #1014, #6487, #11741, #4567, #7329, #9947, #9055, #9001, #10840, #3541, #3717, #4677, #7215, #110, #7446, #3664, #6425, #10899, #11008, #2647, #6312, #8217, #7270, #4620, #8274, #891, #832, #1743, #9886, #5407, #5462, #11073, #4504, #5521, #8157, #2764, #11799, #2884, #10116, #10954, #2711, #3604, #6374, #10000, #1795 ),
 .UNSPECIFIED., .F., .T. ) 
 B_SPLINE_CURVE_WITH_KNOTS ( ( 3, 2, 2, 2, 2, 2, 2, 2, 2, 2, 2, 2, 2, 2, 2, 2, 2, 2, 2, 2, 2, 2, 2, 2, 3 ),
 ( 0.000000000000000000, 0.02083333333333333218, 0.04166666666666666435, 0.06250000000000000000, 0.08333333333333332871, 0.1041666666666666713, 0.1250000000000000000, 0.1458333333333333426, 0.1666666666666666574, 0.1875000000000000000, 0.2083333333333333426, 0.2291666666666666574, 0.2500000000000000000, 0.2708333333333333148, 0.2916666666666666852, 0.3125000000000000000, 0.3333333333333333148, 0.3541666666666666852, 0.3750000000000000000, 0.3958333333333333148, 0.4166666666666666852, 0.4375000000000000000, 0.4583333333333333148, 0.4791666666666666852, 0.4827908099017684251 ),
 .UNSPECIFIED. ) 
 CURVE ( )  GEOMETRIC_REPRESENTATION_ITEM ( )  RATIONAL_B_SPLINE_CURVE ( ( 1.000000000000000000, 0.9238795325112867385, 1.000000000000000000, 0.9238795325112867385, 1.000000000000000000, 0.9238795325112867385, 1.000000000000000000, 0.9238795325112867385, 1.000000000000000000, 0.9238795325112867385, 1.000000000000000000, 0.9238795325112867385, 1.000000000000000000, 0.9238795325112867385, 1.000000000000000000, 0.9238795325112867385, 1.000000000000000000, 0.9238795325112867385, 1.000000000000000000, 0.9238795325112867385, 1.000000000000000000, 0.9238795325112867385, 1.000000000000000000, 0.9238795325112867385, 1.000000000000000000, 0.9238795325112867385, 1.000000000000000000, 0.9238795325112867385, 1.000000000000000000, 0.9238795325112867385, 1.000000000000000000, 0.9238795325112867385, 1.000000000000000000, 0.9238795325112867385, 1.000000000000000000, 0.9238795325112867385, 1.000000000000000000, 0.9238795325112867385, 1.000000000000000000, 0.9238795325112867385, 1.000000000000000000, 0.9238795325112867385, 1.000000000000000000, 0.9238795325112867385, 1.000000000000000000, 0.9238795325112867385, 1.000000000000000000, 0.9867581690895038671, 0.9781234062028126841 ) ) 
 REPRESENTATION_ITEM ( '' )  );
#5546=CARTESIAN_POINT ( 'NONE',  ( -75.96875000204839523, 73.25176868561975141, 18.25176868561974075 ) ) ;
#5552=CARTESIAN_POINT ( 'NONE',  ( -77.93750000000005684, 72.67766952966363192, 17.67766952966363547 ) ) ;
#5575=CARTESIAN_POINT ( 'NONE',  ( -75.21875000204839523, 36.74823131438024859, -18.25176868561973720 ) ) ;
#5585=CARTESIAN_POINT ( 'NONE',  ( -74.99999999999998579, 72.97359286453712457, -18.15706671146198303 ) ) ;
#5589=VECTOR ( 'NONE', #7756, 1000.000000000000000 ) ;
#5591=PRODUCT_DEFINITION_SHAPE ( 'NONE', 'NONE',  #3148 ) ;
#5596=CARTESIAN_POINT ( 'NONE',  ( -72.96875000204838102, 80.81189881250000440, -1.580522963032174394E-15 ) ) ;
#5597=LINE ( 'NONE', #11081, #393 ) ;
#5600=SHAPE_DEFINITION_REPRESENTATION ( #5591, #6185 ) ;
#5616=CARTESIAN_POINT ( 'NONE',  ( -78.31250000000004263, 72.67766952966363192, -17.67766952966363903 ) ) ;
#5639=CARTESIAN_POINT ( 'NONE',  ( -76.90625000204839523, 36.74823131438026280, 18.25176868561974786 ) ) ;
#5649=CARTESIAN_POINT ( 'NONE',  ( -76.71875000409679046, 65.35533905932737753, 24.99999999999999645 ) ) ;
#5662=ADVANCED_FACE ( 'NONE', ( #11287 ), #2249, .F. ) ;
#5680=CARTESIAN_POINT ( 'NONE',  ( -78.12500000409677625, 55.00000000000000000, 24.99999999999999645 ) ) ;
#5683=CARTESIAN_POINT ( 'NONE',  ( -75.87500000409677625, 55.00000000000000000, -24.99999999999999645 ) ) ;
#5700=CARTESIAN_POINT ( 'NONE',  ( -71.65625000204838102, 80.81189881250000440, -1.580522963032174394E-15 ) ) ;
#5709=LINE ( 'NONE', #6672, #8830 ) ;
#5710=CARTESIAN_POINT ( 'NONE',  ( -75.00000000000008527, 62.52349484992671336, -24.64253936146262802 ) ) ;
#5712=CARTESIAN_POINT ( 'NONE',  ( -80.00000000000000000, 55.00000000000000000, -20.00000000000000355 ) ) ;
#5735=ORIENTED_EDGE ( 'NONE', *, *, #2060, .F. ) ;
#5749=CARTESIAN_POINT ( 'NONE',  ( -75.03125000000000000, 80.00000000000001421, 10.35533905932737397 ) ) ;
#5750=CARTESIAN_POINT ( 'NONE',  ( -74.99999999999997158, 56.78048500034128665, -25.76437121692205423 ) ) ;
#5753=CIRCLE ( 'NONE', #566, 29.00000000000000355 ) ;
#5762=CARTESIAN_POINT ( 'NONE',  ( -72.50000000204839523, 29.18810118750000981, 10.69163855873950020 ) ) ;
#5769=CARTESIAN_POINT ( 'NONE',  ( -78.68750000204838102, 44.30836144126052289, 25.81189881250000795 ) ) ;
#5777=CARTESIAN_POINT ( 'NONE',  ( -73.34375000409679046, 30.00000000000001421, 10.35533905932739174 ) ) ;
#5787=ORIENTED_EDGE ( 'NONE', *, *, #6186, .T. ) ;
#5801=CARTESIAN_POINT ( 'NONE',  ( -78.40625000000005684, 65.35533905932518906, -25.00000000000207478 ) ) ;
#5805=CARTESIAN_POINT ( 'NONE',  ( -78.78125000000002842, 30.00000000000003553, -10.35533905932737042 ) ) ;
#5808=CARTESIAN_POINT ( 'NONE',  ( -75.12500000409677625, 55.00000000000000000, 24.99999999999999645 ) ) ;
#5810=CARTESIAN_POINT ( 'NONE',  ( -74.75000000000000000, 55.00000000000000000, 24.99999999999999645 ) ) ;
#5814=DIRECTION ( 'NONE',  ( 0.000000000000000000, 0.000000000000000000, 1.000000000000000000 ) ) ;
#5823=CARTESIAN_POINT ( 'NONE',  ( -78.03125000204839523, 36.74823131438024859, -18.25176868561973720 ) ) ;
#5826=CARTESIAN_POINT ( 'NONE',  ( -76.06250000000005684, 37.32233047033638940, 17.67766952966361771 ) ) ;
#5829=CARTESIAN_POINT ( 'NONE',  ( -78.78125000204838102, 55.00000000000000000, 25.81189881249999729 ) ) ;
#5834=CARTESIAN_POINT ( 'NONE',  ( -72.96875000409677625, 44.64466094067260826, -24.99999999999998934 ) ) ;
#5848=CARTESIAN_POINT ( 'NONE',  ( -76.25000000000000000, 55.00000000000000000, 24.99999999999999645 ) ) ;
#5858=EDGE_CURVE ( 'NONE', #8444, #5404, #8372, .T. ) ;
#5866=CARTESIAN_POINT ( 'NONE',  ( -79.25000000000000000, 55.00000000000000000, 24.99999999999999645 ) ) ;
#5878=CARTESIAN_POINT ( 'NONE',  ( -71.53052368722832455, 77.35376350879521112, 12.90594348738575903 ) ) ;
#5882=FILL_AREA_STYLE_COLOUR ( '', #10845 ) ;
#5885=EDGE_CURVE ( 'NONE', #8444, #4583, #3328, .T. ) ;
#5886=CARTESIAN_POINT ( 'NONE',  ( -80.00000000000000000, 55.00000000000000000, 0.000000000000000000 ) ) ;
#5892=CARTESIAN_POINT ( 'NONE',  ( -72.40625000409677625, 80.00000000000001421, 10.35533905932737397 ) ) ;
#5925=CARTESIAN_POINT ( 'NONE',  ( -76.71875000204839523, 36.74823131438024859, -18.25176868561973720 ) ) ;
#5938=( BOUNDED_SURFACE ( )  B_SPLINE_SURFACE ( 1, 2, ( 
 ( #9049, #6543, #8150, #11735, #5514, #9103, #7207, #42, #11790, #1736, #7373, #6306, #11000, #7263, #9161, #9994, #10892, #10832, #2876, #5401, #2639, #3535, #4612, #2702, #1789, #6368, #4558, #8268, #8208, #10948, #945, #6480, #11844, #1009, #10173, #2758, #8099, #6418, #11065, #10048, #5342, #1846, #3710, #2812, #3770, #10107, #5575, #9221, #4669, #8994, #769, #4446, #9520, #166, #4014, #4916, #3117, #9399, #3837, #2152, #2936, #7732, #1127, #11307, #11125, #11363, #8629, #1067, #4795, #2210, #10294, #10232, #1311, #3895, #4733, #5762, #9460, #9338, #8451, #10412, #2026, #7672, #3952, #6605, #5700, #231, #5878 ),
 ( #7557, #4977, #1194, #410, #11180, #2994, #8387, #7614, #7501, #9274, #6661, #4075, #2088, #3054, #5823, #288, #4858, #8508, #1969, #11243, #3172, #6724, #10355, #1246, #8568, #6840, #5639, #347, #6783, #525, #11417, #10635, #6059, #2383, #3288, #6957, #10524, #2332, #11659, #9636, #5039, #2448, #9694, #468, #5212, #1432, #6896, #641, #3228, #4303, #5095, #6114, #10583, #8742, #4125, #8021, #6003, #7788, #8686, #9748, #4186, #1491, #7848, #11476, #1545, #5151, #582, #8862, #11596, #8803, #6176, #3469, #4249, #1376, #7908, #4369, #11537, #10466, #3341, #7012, #7961, #8915, #3402, #7075, #10700, #2512, #9806 ) ),
 .UNSPECIFIED., .F., .F., .T. ) 
 B_SPLINE_SURFACE_WITH_KNOTS ( ( 2, 2 ),
 ( 3, 2, 2, 2, 2, 2, 2, 2, 2, 2, 2, 2, 2, 2, 2, 2, 2, 2, 2, 2, 2, 2, 2, 2, 2, 2, 2, 2, 2, 2, 2, 2, 2, 2, 2, 2, 2, 2, 2, 2, 2, 2, 2, 3 ),
 ( 0.000000000000000000, 1.000000000000000000 ),
 ( 0.000000000000000000, 0.02083333333333333218, 0.04166666666666666435, 0.06250000000000000000, 0.08333333333333332871, 0.1041666666666666713, 0.1250000000000000000, 0.1458333333333333426, 0.1666666666666666574, 0.1875000000000000000, 0.2083333333333333426, 0.2291666666666666574, 0.2500000000000000000, 0.2708333333333333148, 0.2916666666666666852, 0.3125000000000000000, 0.3333333333333333148, 0.3541666666666666852, 0.3750000000000000000, 0.3958333333333333148, 0.4166666666666666852, 0.4375000000000000000, 0.4583333333333333148, 0.4791666666666666852, 0.5000000000000000000, 0.5208333333333333703, 0.5416666666666666297, 0.5625000000000000000, 0.5833333333333333703, 0.6041666666666666297, 0.6250000000000000000, 0.6458333333333333703, 0.6666666666666666297, 0.6875000000000000000, 0.7083333333333333703, 0.7291666666666666297, 0.7500000000000000000, 0.7708333333333333703, 0.7916666666666666297, 0.8125000000000000000, 0.8333333333333333703, 0.8541666666666666297, 0.8750000000000000000, 0.8888490476107191451 ),
 .UNSPECIFIED. ) 
 GEOMETRIC_REPRESENTATION_ITEM ( )  RATIONAL_B_SPLINE_SURFACE ( (
 ( 1.000000000000000000, 0.9238795325112867385, 1.000000000000000000, 0.9238795325112867385, 1.000000000000000000, 0.9238795325112867385, 1.000000000000000000, 0.9238795325112867385, 1.000000000000000000, 0.9238795325112867385, 1.000000000000000000, 0.9238795325112867385, 1.000000000000000000, 0.9238795325112867385, 1.000000000000000000, 0.9238795325112867385, 1.000000000000000000, 0.9238795325112867385, 1.000000000000000000, 0.9238795325112867385, 1.000000000000000000, 0.9238795325112867385, 1.000000000000000000, 0.9238795325112867385, 1.000000000000000000, 0.9238795325112867385, 1.000000000000000000, 0.9238795325112867385, 1.000000000000000000, 0.9238795325112867385, 1.000000000000000000, 0.9238795325112867385, 1.000000000000000000, 0.9238795325112867385, 1.000000000000000000, 0.9238795325112867385, 1.000000000000000000, 0.9238795325112867385, 1.000000000000000000, 0.9238795325112867385, 1.000000000000000000, 0.9238795325112867385, 1.000000000000000000, 0.9238795325112867385, 1.000000000000000000, 0.9238795325112867385, 1.000000000000000000, 0.9238795325112867385, 1.000000000000000000, 0.9238795325112867385, 1.000000000000000000, 0.9238795325112867385, 1.000000000000000000, 0.9238795325112867385, 1.000000000000000000, 0.9238795325112867385, 1.000000000000000000, 0.9238795325112867385, 1.000000000000000000, 0.9238795325112867385, 1.000000000000000000, 0.9238795325112867385, 1.000000000000000000, 0.9238795325112867385, 1.000000000000000000, 0.9238795325112867385, 1.000000000000000000, 0.9238795325112867385, 1.000000000000000000, 0.9238795325112867385, 1.000000000000000000, 0.9238795325112867385, 1.000000000000000000, 0.9238795325112867385, 1.000000000000000000, 0.9238795325112867385, 1.000000000000000000, 0.9238795325112867385, 1.000000000000000000, 0.9238795325112867385, 1.000000000000000000, 0.9238795325112867385, 1.000000000000000000, 0.9238795325112867385, 1.000000000000000000, 0.9493985930367334625, 0.9660721903170175207),
 ( 1.000000000000000000, 0.9238795325112867385, 1.000000000000000000, 0.9238795325112867385, 1.000000000000000000, 0.9238795325112867385, 1.000000000000000000, 0.9238795325112867385, 1.000000000000000000, 0.9238795325112867385, 1.000000000000000000, 0.9238795325112867385, 1.000000000000000000, 0.9238795325112867385, 1.000000000000000000, 0.9238795325112867385, 1.000000000000000000, 0.9238795325112867385, 1.000000000000000000, 0.9238795325112867385, 1.000000000000000000, 0.9238795325112867385, 1.000000000000000000, 0.9238795325112867385, 1.000000000000000000, 0.9238795325112867385, 1.000000000000000000, 0.9238795325112867385, 1.000000000000000000, 0.9238795325112867385, 1.000000000000000000, 0.9238795325112867385, 1.000000000000000000, 0.9238795325112867385, 1.000000000000000000, 0.9238795325112867385, 1.000000000000000000, 0.9238795325112867385, 1.000000000000000000, 0.9238795325112867385, 1.000000000000000000, 0.9238795325112867385, 1.000000000000000000, 0.9238795325112867385, 1.000000000000000000, 0.9238795325112867385, 1.000000000000000000, 0.9238795325112867385, 1.000000000000000000, 0.9238795325112867385, 1.000000000000000000, 0.9238795325112867385, 1.000000000000000000, 0.9238795325112867385, 1.000000000000000000, 0.9238795325112867385, 1.000000000000000000, 0.9238795325112867385, 1.000000000000000000, 0.9238795325112867385, 1.000000000000000000, 0.9238795325112867385, 1.000000000000000000, 0.9238795325112867385, 1.000000000000000000, 0.9238795325112867385, 1.000000000000000000, 0.9238795325112867385, 1.000000000000000000, 0.9238795325112867385, 1.000000000000000000, 0.9238795325112867385, 1.000000000000000000, 0.9238795325112867385, 1.000000000000000000, 0.9238795325112867385, 1.000000000000000000, 0.9238795325112867385, 1.000000000000000000, 0.9238795325112867385, 1.000000000000000000, 0.9238795325112867385, 1.000000000000000000, 0.9238795325112867385, 1.000000000000000000, 0.9493985930367334625, 0.9660721903170175207) ) ) 
 REPRESENTATION_ITEM ( '' )  SURFACE ( )  );
#5945=CARTESIAN_POINT ( 'NONE',  ( -75.87500000000007105, 30.00000000000010303, 4.592425496802555434E-15 ) ) ;
#5946=( NAMED_UNIT ( * ) SI_UNIT ( $, .STERADIAN. ) SOLID_ANGLE_UNIT ( ) );
#5957=ADVANCED_FACE ( 'NONE', ( #1401 ), #1411, .T. ) ;
#5965=EDGE_CURVE ( 'NONE', #7521, #10082, #5753, .T. ) ;
#5991=CARTESIAN_POINT ( 'NONE',  ( -72.96875000000000000, 30.00000000000001421, 10.35533905932739174 ) ) ;
#6003=CARTESIAN_POINT ( 'NONE',  ( -74.09375000204839523, 55.00000000000000000, 25.81189881249999729 ) ) ;
#6011=( BOUNDED_CURVE ( )  B_SPLINE_CURVE ( 2, ( #897, #3609, #7829, #8723, #11805, #5412, #8110, #6942, #7276 ),
 .UNSPECIFIED., .F., .T. ) 
 B_SPLINE_CURVE_WITH_KNOTS ( ( 3, 2, 2, 2, 3 ),
 ( 0.2500000000000002220, 0.2708333333333335369, 0.2916666666666669627, 0.3125000000000002776, 0.3333333333333335924 ),
 .UNSPECIFIED. ) 
 CURVE ( )  GEOMETRIC_REPRESENTATION_ITEM ( )  RATIONAL_B_SPLINE_CURVE ( ( 0.9999999999999992228, 0.9238795325112875156, 1.000000000000000000, 0.9238795325112867385, 1.000000000000000000, 0.9238795325112867385, 1.000000000000000000, 0.9238795325112857393, 1.000000000000001110 ) ) 
 REPRESENTATION_ITEM ( '' )  );
#6020=CARTESIAN_POINT ( 'NONE',  ( -78.31250000409679046, 72.67766952966368876, 17.67766952966368521 ) ) ;
#6027=CARTESIAN_POINT ( 'NONE',  ( -75.21875000204839523, 29.18810118750000271, 4.741568889096522788E-15 ) ) ;
#6029=CARTESIAN_POINT ( 'NONE',  ( -75.06471690546626974, 79.99999999999991473, 6.658686756724147671 ) ) ;
#6033=CARTESIAN_POINT ( 'NONE',  ( -75.00000000000002842, 31.34658496415306672, -9.793415029090784429 ) ) ;
#6041=CARTESIAN_POINT ( 'NONE',  ( -79.25000000000000000, 55.00000000000000000, 24.99999999999999645 ) ) ;
#6045=CARTESIAN_POINT ( 'NONE',  ( -78.12500000204838102, 44.30836144126050158, -25.81189881249999374 ) ) ;
#6047=PRODUCT_DEFINITION_FORMATION_WITH_SPECIFIED_SOURCE ( 'ANY', '', #1748, .NOT_KNOWN. ) ;
#6048=CARTESIAN_POINT ( 'NONE',  ( -75.00000000000000000, 55.00000000000000000, 0.000000000000000000 ) ) ;
#6054=CYLINDRICAL_SURFACE ( 'NONE', #11001, 20.00000000000000355 ) ;
#6059=CARTESIAN_POINT ( 'NONE',  ( -76.34375000204839523, 55.00000000000000000, -25.81189881249999729 ) ) ;
#6060=ORIENTED_EDGE ( 'NONE', *, *, #5885, .F. ) ;
#6066=CARTESIAN_POINT ( 'NONE',  ( -76.15625000204838102, 80.81189881250000440, -1.580522963032174394E-15 ) ) ;
#6085=CARTESIAN_POINT ( 'NONE',  ( -78.87500000204838102, 80.81189881250001861, 10.69163855873948599 ) ) ;
#6092=EDGE_LOOP ( 'NONE', ( #2547, #5229, #9215 ) ) ;
#6103=CARTESIAN_POINT ( 'NONE',  ( -78.50000000204840944, 29.18810118750000981, 10.69163855873950020 ) ) ;
#6111=CARTESIAN_POINT ( 'NONE',  ( -83.00000000000000000, 55.00000000000000000, 0.000000000000000000 ) ) ;
#6113=DIRECTION ( 'NONE',  ( 0.000000000000000000, 0.000000000000000000, 1.000000000000000000 ) ) ;
#6114=CARTESIAN_POINT ( 'NONE',  ( -74.56250000204839523, 80.81189881250001861, -10.69163855873949132 ) ) ;
#6122=CARTESIAN_POINT ( 'NONE',  ( -77.00000000204839523, 29.18810118750000981, 10.69163855873950020 ) ) ;
#6124=DIRECTION ( 'NONE',  ( -1.000000000000000000, 0.000000000000000000, 0.000000000000000000 ) ) ;
#6142=CARTESIAN_POINT ( 'NONE',  ( -75.68750000204839523, 65.69163855873949842, 25.81189881250000440 ) ) ;
#6162=CARTESIAN_POINT ( 'NONE',  ( -77.09375000204839523, 36.74823131438026280, 18.25176868561974786 ) ) ;
#6164=CARTESIAN_POINT ( 'NONE',  ( 0.000000000000000000, 0.000000000000000000, 0.000000000000000000 ) ) ;
#6176=CARTESIAN_POINT ( 'NONE',  ( -72.78125000204839523, 73.25176868561975141, 18.25176868561974075 ) ) ;
#6184=CARTESIAN_POINT ( 'NONE',  ( -78.03125000204838102, 55.00000000000000000, -25.81189881249999729 ) ) ;
#6185=SHAPE_REPRESENTATION ( 'Threaded Front Retaining Ring Collar', ( #4738 ), #3395 ) ;
#6186=EDGE_CURVE ( 'NONE', #10943, #4583, #370, .T. ) ;
#6198=CARTESIAN_POINT ( 'NONE',  ( -78.68750000409679046, 72.67766952966368876, -17.67766952966368876 ) ) ;
#6204=CARTESIAN_POINT ( 'NONE',  ( -77.56250000204839523, 80.81189881250001861, -10.69163855873949132 ) ) ;
#6209=ORIENTED_EDGE ( 'NONE', *, *, #4119, .T. ) ;
#6218=CARTESIAN_POINT ( 'NONE',  ( -74.09375000204839523, 36.74823131438026280, 18.25176868561974786 ) ) ;
#6220=( LENGTH_UNIT ( ) NAMED_UNIT ( * ) SI_UNIT ( .MILLI., .METRE. ) );
#6227=ORIENTED_EDGE ( 'NONE', *, *, #6469, .F. ) ;
#6257=CARTESIAN_POINT ( 'NONE',  ( -78.78125000409680467, 65.35533905932737753, -24.99999999999999645 ) ) ;
#6258=CARTESIAN_POINT ( 'NONE',  ( -83.00000000000000000, 55.00000000000000000, 20.00000000000000355 ) ) ;
#6264=CARTESIAN_POINT ( 'NONE',  ( -74.00000000204840944, 44.30836144126053000, 25.81189881250000795 ) ) ;
#6277=CARTESIAN_POINT ( 'NONE',  ( -75.00000000000000000, 55.00000000000000000, 25.00000000000000355 ) ) ;
#6280=CARTESIAN_POINT ( 'NONE',  ( -72.59375000204838102, 36.74823131438026280, 18.25176868561974786 ) ) ;
#6306=CARTESIAN_POINT ( 'NONE',  ( -78.50000000204840944, 29.18810118750000981, 10.69163855873950020 ) ) ;
#6312=CARTESIAN_POINT ( 'NONE',  ( -77.09375000204839523, 55.00000000000000000, 25.81189881249999729 ) ) ;
#6314=ADVANCED_FACE ( 'NONE', ( #9939 ), #5938, .T. ) ;
#6321=CARTESIAN_POINT ( 'NONE',  ( -75.96875000409677625, 44.64466094067260826, -24.99999999999998934 ) ) ;
#6328=AXIS2_PLACEMENT_3D ( 'NONE', #4320, #5228, #11494 ) ;
#6336=ORIENTED_EDGE ( 'NONE', *, *, #3731, .F. ) ;
#6337=CARTESIAN_POINT ( 'NONE',  ( -74.46875000204839523, 73.25176868561975141, 18.25176868561974075 ) ) ;
#6344=ORIENTED_EDGE ( 'NONE', *, *, #2060, .T. ) ;
#6347=AXIS2_PLACEMENT_3D ( 'NONE', #3248, #3490, #10550 ) ;
#6368=CARTESIAN_POINT ( 'NONE',  ( -77.18750000204838102, 44.30836144126053000, 25.81189881250000795 ) ) ;
#6369=ORIENTED_EDGE ( 'NONE', *, *, #3354, .F. ) ;
#6374=CARTESIAN_POINT ( 'NONE',  ( -75.03125000204839523, 36.74823131438024859, -18.25176868561973720 ) ) ;
#6376=FACE_OUTER_BOUND ( 'NONE', #7651, .T. ) ;
#6379=CARTESIAN_POINT ( 'NONE',  ( -77.37500000409677625, 55.00000000000000000, -24.99999999999999645 ) ) ;
#6392=CARTESIAN_POINT ( 'NONE',  ( -75.21875000204839523, 36.74823131438024859, -18.25176868561973720 ) ) ;
#6403=CARTESIAN_POINT ( 'NONE',  ( -80.00000000000000000, 55.00000000000000000, 0.000000000000000000 ) ) ;
#6418=CARTESIAN_POINT ( 'NONE',  ( -76.06250000204839523, 80.81189881250001861, 10.69163855873948599 ) ) ;
#6425=CARTESIAN_POINT ( 'NONE',  ( -77.46875000204839523, 80.81189881250000440, -1.580522963032174394E-15 ) ) ;
#6431=CARTESIAN_POINT ( 'NONE',  ( -72.50000000204839523, 44.30836144126053000, 25.81189881250000795 ) ) ;
#6447=CARTESIAN_POINT ( 'NONE',  ( -76.06250000204839523, 80.81189881250001861, 10.69163855873948599 ) ) ;
#6453=EDGE_CURVE ( 'NONE', #5404, #5247, #9979, .T. ) ;
#6463=DIRECTION ( 'NONE',  ( -1.000000000000000000, 0.000000000000000000, 0.000000000000000000 ) ) ;
#6469=EDGE_CURVE ( 'NONE', #11373, #11066, #3448, .T. ) ;
#6478=CARTESIAN_POINT ( 'NONE',  ( -83.00000000000000000, 55.00000000000000000, -20.00000000000000355 ) ) ;
#6480=CARTESIAN_POINT ( 'NONE',  ( -76.62500000204839523, 44.30836144126050158, -25.81189881249999374 ) ) ;
#6487=CARTESIAN_POINT ( 'NONE',  ( -78.87500000204839523, 80.81189881250000440, 10.69163855873948243 ) ) ;
#6488=CARTESIAN_POINT ( 'NONE',  ( -75.00000000000001421, 70.68788533342120672, -20.24596063305270377 ) ) ;
#6492=CARTESIAN_POINT ( 'NONE',  ( -71.46875000204838102, 80.81189881250000440, -1.580522963032174394E-15 ) ) ;
#6493=VECTOR ( 'NONE', #459, 1000.000000000000000 ) ;
#6525=CARTESIAN_POINT ( 'NONE',  ( -75.31250000000007105, 72.67766952966361771, -17.67766952966361416 ) ) ;
#6543=CARTESIAN_POINT ( 'NONE',  ( -79.43750000204838102, 65.69163855873948421, -25.81189881250000440 ) ) ;
#6554=CARTESIAN_POINT ( 'NONE',  ( -75.00000000000001421, 80.21963981261983179, 0.1224285101258584668 ) ) ;
#6558=ORIENTED_EDGE ( 'NONE', *, *, #1321, .T. ) ;
#6560=CARTESIAN_POINT ( 'NONE',  ( -72.12500000204840944, 29.18810118750000626, -10.69163855873949309 ) ) ;
#6590=CARTESIAN_POINT ( 'NONE',  ( -79.34375000000002842, 65.35533905932737753, 24.99999999999999645 ) ) ;
#6605=CARTESIAN_POINT ( 'NONE',  ( -71.75000000204838102, 80.81189881250001861, -10.69163855873949132 ) ) ;
#6612=CARTESIAN_POINT ( 'NONE',  ( -75.00000000000004263, 60.52393795488850969, -25.20097221523710473 ) ) ;
#6616=CARTESIAN_POINT ( 'NONE',  ( -71.65625000409677625, 30.00000000000000355, -10.35533905932738108 ) ) ;
#6618=CARTESIAN_POINT ( 'NONE',  ( -78.50000000000000000, 55.00000000000000000, -24.99999999999999645 ) ) ;
#6631=CARTESIAN_POINT ( 'NONE',  ( -76.34375000000005684, 65.35533905932732068, 24.99999999999990052 ) ) ;
#6645=CARTESIAN_POINT ( 'NONE',  ( -75.40625000409677625, 80.00000000000001421, 10.35533905932737397 ) ) ;
#6647=CARTESIAN_POINT ( 'NONE',  ( -75.21875000000000000, 80.00000000000001421, -10.35533905932737753 ) ) ;
#6659=EDGE_CURVE ( 'NONE', #8886, #879, #176, .T. ) ;
#6661=CARTESIAN_POINT ( 'NONE',  ( -78.40625000204839523, 36.74823131438026280, 18.25176868561974786 ) ) ;
#6664=EDGE_CURVE ( 'NONE', #9420, #9375, #9600, .T. ) ;
#6667=ORIENTED_EDGE ( 'NONE', *, *, #5858, .T. ) ;
#6669=STYLED_ITEM ( 'NONE', ( #8905 ), #7857 ) ;
#6672=CARTESIAN_POINT ( 'NONE',  ( -75.00000000000000000, 55.00000000000000000, -25.00000000000000355 ) ) ;
#6673=CARTESIAN_POINT ( 'NONE',  ( -75.00000000000002842, 69.01357686183018814, -21.46027625722670606 ) ) ;
#6678=CARTESIAN_POINT ( 'NONE',  ( -74.75000000409677625, 30.00000000000000355, 4.592425496802573578E-15 ) ) ;
#6712=CARTESIAN_POINT ( 'NONE',  ( -78.59375000000001421, 44.64466094067260826, -24.99999999999998934 ) ) ;
#6724=CARTESIAN_POINT ( 'NONE',  ( -77.37500000204838102, 80.81189881250001861, 10.69163855873948599 ) ) ;
#6772=CARTESIAN_POINT ( 'NONE',  ( -79.81250000000001421, 72.67766952966368876, -17.67766952966368876 ) ) ;
#6783=CARTESIAN_POINT ( 'NONE',  ( -76.71875000204839523, 29.18810118750000271, 4.741568889096522788E-15 ) ) ;
#6788=CARTESIAN_POINT ( 'NONE',  ( -78.31250000204838102, 29.18810118750000626, -10.69163855873949132 ) ) ;
#6795=CARTESIAN_POINT ( 'NONE',  ( -74.37500000409677625, 55.00000000000000000, -24.99999999999999645 ) ) ;
#6825=CARTESIAN_POINT ( 'NONE',  ( -78.50000000000000000, 55.00000000000000000, -24.99999999999999645 ) ) ;
#6840=CARTESIAN_POINT ( 'NONE',  ( -77.00000000204838102, 44.30836144126053000, 25.81189881250000795 ) ) ;
#6857=CARTESIAN_POINT ( 'NONE',  ( -73.81250000409677625, 72.67766952966368876, 17.67766952966368521 ) ) ;
#6883=CARTESIAN_POINT ( 'NONE',  ( -76.62500000204839523, 44.30836144126050158, -25.81189881249999374 ) ) ;
#6884=CARTESIAN_POINT ( 'NONE',  ( -75.00000000000001421, 51.71064787084756631, -25.65688961934584356 ) ) ;
#6896=CARTESIAN_POINT ( 'NONE',  ( -75.03125000204839523, 36.74823131438024859, -18.25176868561973720 ) ) ;
#6904=CARTESIAN_POINT ( 'NONE',  ( -76.06250000204839523, 80.81189881250000440, 10.69163855873948243 ) ) ;
#6909=CARTESIAN_POINT ( 'NONE',  ( -79.34375000204839523, 55.00000000000000000, -25.81189881249999729 ) ) ;
#6927=CARTESIAN_POINT ( 'NONE',  ( -73.62500000204842365, 29.18810118750000626, -10.69163855873949309 ) ) ;
#6928=CARTESIAN_POINT ( 'NONE',  ( -75.59375000409677625, 80.00000000000001421, -10.35533905932737753 ) ) ;
#6942=CARTESIAN_POINT ( 'NONE',  ( -75.96875000409676204, 44.64466094067271484, -25.00000000000010303 ) ) ;
#6945=CARTESIAN_POINT ( 'NONE',  ( -78.31250000204838102, 29.18810118750000626, -10.69163855873949309 ) ) ;
#6957=CARTESIAN_POINT ( 'NONE',  ( -76.06250000204840944, 80.81189881250001861, -10.69163855873949132 ) ) ;
#6964=CARTESIAN_POINT ( 'NONE',  ( -76.81250000204838102, 29.18810118750000626, -10.69163855873949132 ) ) ;
#6976=FACE_BOUND ( 'NONE', #3507, .T. ) ;
#6984=CARTESIAN_POINT ( 'NONE',  ( -77.84375000204839523, 55.00000000000000000, -25.81189881249999729 ) ) ;
#6999=CARTESIAN_POINT ( 'NONE',  ( -73.15625000000000000, 44.64466094067262958, 25.00000000000001066 ) ) ;
#7001=EDGE_LOOP ( 'NONE', ( #3440, #7476 ) ) ;
#7012=CARTESIAN_POINT ( 'NONE',  ( -71.93750000204838102, 44.30836144126050158, -25.81189881249999374 ) ) ;
#7020=CARTESIAN_POINT ( 'NONE',  ( -76.71875000204839523, 36.74823131438024859, -18.25176868561973720 ) ) ;
#7046=CARTESIAN_POINT ( 'NONE',  ( -76.15625000204839523, 73.25176868561975141, -18.25176868561974430 ) ) ;
#7062=CARTESIAN_POINT ( 'NONE',  ( -79.06250000204839523, 80.81189881250001861, 10.69163855873948599 ) ) ;
#7075=CARTESIAN_POINT ( 'NONE',  ( -71.56250000204838102, 80.81189881250001861, -10.69163855873949132 ) ) ;
#7081=AXIS2_PLACEMENT_3D ( 'NONE', #8133, #9922, #6113 ) ;
#7083=CARTESIAN_POINT ( 'NONE',  ( -75.01598058408755776, 56.74138771028714956, -25.81189881249999729 ) ) ;
#7088=LINE ( 'NONE', #10539, #7512 ) ;
#7103=CARTESIAN_POINT ( 'NONE',  ( -79.25000000204838102, 65.69163855873948421, -25.81189881250000440 ) ) ;
#7107=CARTESIAN_POINT ( 'NONE',  ( -77.00000000409677625, 80.00000000000000000, -1.530808498934191324E-15 ) ) ;
#7122=CARTESIAN_POINT ( 'NONE',  ( -77.46875000204839523, 73.25176868561975141, 18.25176868561974075 ) ) ;
#7125=EDGE_CURVE ( 'NONE', #7495, #10833, #5597, .T. ) ;
#7141=EDGE_LOOP ( 'NONE', ( #11818, #8452, #7956, #5307 ) ) ;
#7146=CARTESIAN_POINT ( 'NONE',  ( -83.00000000000000000, 55.00000000000000000, 0.000000000000000000 ) ) ;
#7159=ORIENTED_EDGE ( 'NONE', *, *, #9027, .T. ) ;
#7161=CARTESIAN_POINT ( 'NONE',  ( -75.03125000204839523, 36.74823131438024859, -18.25176868561973720 ) ) ;
#7166=CARTESIAN_POINT ( 'NONE',  ( -74.99999999999997158, 35.03849855854433315, 15.32554794922328156 ) ) ;
#7175=CARTESIAN_POINT ( 'NONE',  ( -74.56250000204839523, 80.81189881250001861, 10.69163855873948599 ) ) ;
#7178=ADVANCED_FACE ( 'NONE', ( #363 ), #7745, .F. ) ;
#7187=DIRECTION ( 'NONE',  ( -1.000000000000000000, 0.000000000000000000, 0.000000000000000000 ) ) ;
#7207=CARTESIAN_POINT ( 'NONE',  ( -78.96875000204839523, 73.25176868561975141, 18.25176868561974075 ) ) ;
#7215=CARTESIAN_POINT ( 'NONE',  ( -77.84375000204839523, 55.00000000000000000, -25.81189881249999729 ) ) ;
#7222=CARTESIAN_POINT ( 'NONE',  ( -72.68750000204839523, 65.69163855873949842, 25.81189881250000440 ) ) ;
#7239=CARTESIAN_POINT ( 'NONE',  ( -71.48947498017410851, 75.17259594761931396, 16.68383898576512081 ) ) ;
#7263=CARTESIAN_POINT ( 'NONE',  ( -78.31250000204838102, 29.18810118750000626, -10.69163855873949309 ) ) ;
#7266=ORIENTED_EDGE ( 'NONE', *, *, #9234, .T. ) ;
#7270=CARTESIAN_POINT ( 'NONE',  ( -76.90625000204839523, 36.74823131438026280, 18.25176868561974786 ) ) ;
#7276=CARTESIAN_POINT ( 'NONE',  ( -75.87500000409677625, 55.00000000000000000, -24.99999999999999645 ) ) ;
#7277=CARTESIAN_POINT ( 'NONE',  ( -71.84375000204838102, 55.00000000000000000, -25.81189881249999729 ) ) ;
#7292=CARTESIAN_POINT ( 'NONE',  ( -72.78125000204838102, 55.00000000000000000, 25.81189881249999729 ) ) ;
#7313=CARTESIAN_POINT ( 'NONE',  ( -80.00000000000000000, 55.00000000000000000, 25.00000000000000355 ) ) ;
#7323=ORIENTED_EDGE ( 'NONE', *, *, #6453, .T. ) ;
#7329=CARTESIAN_POINT ( 'NONE',  ( -78.59375000204839523, 55.00000000000000000, 25.81189881249999729 ) ) ;
#7334=CARTESIAN_POINT ( 'NONE',  ( -75.03125000409677625, 44.64466094067262958, 25.00000000000001066 ) ) ;
#7350=CARTESIAN_POINT ( 'NONE',  ( -73.43750000204839523, 65.69163855873948421, -25.81189881250000440 ) ) ;
#7359=FACE_OUTER_BOUND ( 'NONE', #1470, .T. ) ;
#7373=CARTESIAN_POINT ( 'NONE',  ( -78.59375000204839523, 36.74823131438026280, 18.25176868561974786 ) ) ;
#7383=CARTESIAN_POINT ( 'NONE',  ( -75.00000000000000000, 69.43970489681053948, -21.16564186330591468 ) ) ;
#7387=CARTESIAN_POINT ( 'NONE',  ( -71.40810441781462714, 80.81189881250000440, 6.916273779317701376 ) ) ;
#7394=( BOUNDED_CURVE ( )  B_SPLINE_CURVE ( 2, ( #689, #8013, #11651, #8343, #1932, #1991, #10377, #129, #3793 ),
 .UNSPECIFIED., .F., .T. ) 
 B_SPLINE_CURVE_WITH_KNOTS ( ( 3, 2, 2, 2, 3 ),
 ( 0.000000000000000000, 0.01979916996583446290, 0.03959833993166892580, 0.05939750989750339216, 0.07919667986333785159 ),
 .UNSPECIFIED. ) 
 CURVE ( )  GEOMETRIC_REPRESENTATION_ITEM ( )  RATIONAL_B_SPLINE_CURVE ( ( 1.000000000000000000, 0.9238795325112868495, 1.000000000000000000, 0.9238795325112868495, 1.000000000000000000, 0.9238795325112868495, 1.000000000000000000, 0.9238795325112868495, 1.000000000000000000 ) ) 
 REPRESENTATION_ITEM ( '' )  );
#7399=ORIENTED_EDGE ( 'NONE', *, *, #1321, .F. ) ;
#7404=CARTESIAN_POINT ( 'NONE',  ( -71.53052369147286527, 77.35376373433385311, 12.90594309674112949 ) ) ;
#7412=CARTESIAN_POINT ( 'NONE',  ( -77.84374999999997158, 65.35533905932209109, 25.00000000000518341 ) ) ;
#7446=CARTESIAN_POINT ( 'NONE',  ( -77.65625000204839523, 73.25176868561975141, -18.25176868561974430 ) ) ;
#7448=CARTESIAN_POINT ( 'NONE',  ( -74.99999999999997158, 79.03756697387808572, 7.232545519770552822 ) ) ;
#7452=CARTESIAN_POINT ( 'NONE',  ( -72.21875000204838102, 29.18810118750000271, 4.741568889096522788E-15 ) ) ;
#7453=AXIS2_PLACEMENT_3D ( 'NONE', #6048, #2502, #2319 ) ;
#7457=PRODUCT_CONTEXT ( 'NONE', #4944, 'mechanical' ) ;
#7459=AXIS2_PLACEMENT_3D ( 'NONE', #6403, #10872, #4540 ) ;
#7470=VECTOR ( 'NONE', #7598, 1000.000000000000000 ) ;
#7476=ORIENTED_EDGE ( 'NONE', *, *, #7559, .T. ) ;
#7483=DIRECTION ( 'NONE',  ( 0.000000000000000000, 0.000000000000000000, 1.000000000000000000 ) ) ;
#7488=CARTESIAN_POINT ( 'NONE',  ( -78.78125000000001421, 30.00000000000000355, -10.35533905932738108 ) ) ;
#7495=VERTEX_POINT ( 'NONE', #1660 ) ;
#7501=CARTESIAN_POINT ( 'NONE',  ( -78.59375000204839523, 55.00000000000000000, 25.81189881249999729 ) ) ;
#7512=VECTOR ( 'NONE', #4537, 1000.000000000000000 ) ;
#7515=CARTESIAN_POINT ( 'NONE',  ( -71.93750000409677625, 37.32233047033631124, 17.67766952966369232 ) ) ;
#7521=VERTEX_POINT ( 'NONE', #1777 ) ;
#7539=CARTESIAN_POINT ( 'NONE',  ( -77.84375000409677625, 30.00000000000001421, 10.35533905932739174 ) ) ;
#7548=CARTESIAN_POINT ( 'NONE',  ( -83.00000000000000000, 55.00000000000000711, -29.00000000000000355 ) ) ;
#7557=CARTESIAN_POINT ( 'NONE',  ( -79.34375000204839523, 55.00000000000000000, -25.81189881249999729 ) ) ;
#7559=EDGE_CURVE ( 'NONE', #9652, #2004, #9587, .T. ) ;
#7571=CARTESIAN_POINT ( 'NONE',  ( -71.37500000409677625, 55.00000000000000000, -24.99999999999999645 ) ) ;
#7578=DIRECTION ( 'NONE',  ( 0.000000000000000000, 0.000000000000000000, 1.000000000000000000 ) ) ;
#7598=DIRECTION ( 'NONE',  ( 1.000000000000000000, 0.000000000000000000, 0.000000000000000000 ) ) ;
#7601=CARTESIAN_POINT ( 'NONE',  ( -75.40625000000000000, 65.35533905932737753, -24.99999999999999645 ) ) ;
#7614=CARTESIAN_POINT ( 'NONE',  ( -78.68750000204839523, 65.69163855873949842, 25.81189881250000440 ) ) ;
#7622=CARTESIAN_POINT ( 'NONE',  ( -75.00000000000000000, 80.20344453945780572, -1.438425885725281628 ) ) ;
#7639=ORIENTED_EDGE ( 'NONE', *, *, #4379, .F. ) ;
#7642=CARTESIAN_POINT ( 'NONE',  ( -76.43750000000005684, 72.67766952966361771, 17.67766952966361771 ) ) ;
#7651=EDGE_LOOP ( 'NONE', ( #10816, #420, #10108, #6369 ) ) ;
#7654=CARTESIAN_POINT ( 'NONE',  ( -78.68750000000002842, 37.32233047033633966, -17.67766952966366034 ) ) ;
#7660=CARTESIAN_POINT ( 'NONE',  ( -77.46875000000000000, 30.00000000000001421, 10.35533905932739174 ) ) ;
#7669=LINE ( 'NONE', #3225, #9832 ) ;
#7672=CARTESIAN_POINT ( 'NONE',  ( -71.93750000204838102, 65.69163855873948421, -25.81189881250000440 ) ) ;
#7679=CARTESIAN_POINT ( 'NONE',  ( -78.59375000204839523, 36.74823131438026280, 18.25176868561974786 ) ) ;
#7712=ADVANCED_FACE ( 'NONE', ( #10280 ), #3864, .T. ) ;
#7718=EDGE_CURVE ( 'NONE', #7495, #2377, #11189, .T. ) ;
#7720=CYLINDRICAL_SURFACE ( 'NONE', #3436, 25.00000000000000355 ) ;
#7722=CARTESIAN_POINT ( 'NONE',  ( -75.59375000000000000, 44.64466094067260826, -24.99999999999998934 ) ) ;
#7732=CARTESIAN_POINT ( 'NONE',  ( -73.81250000204839523, 29.18810118750000626, -10.69163855873949309 ) ) ;
#7738=CARTESIAN_POINT ( 'NONE',  ( -78.12500000204839523, 44.30836144126049447, -25.81189881249999019 ) ) ;
#7740=CARTESIAN_POINT ( 'NONE',  ( -75.00000000000000000, 55.00000000000000000, 0.000000000000000000 ) ) ;
#7744=CARTESIAN_POINT ( 'NONE',  ( -71.00000000409677625, 80.00000000000000000, -1.530808498934191324E-15 ) ) ;
#7745=CYLINDRICAL_SURFACE ( 'NONE', #4233, 25.00000000000000355 ) ;
#7756=DIRECTION ( 'NONE',  ( -1.000000000000000000, 0.000000000000000000, 0.000000000000000000 ) ) ;
#7757=CARTESIAN_POINT ( 'NONE',  ( -78.87500000409677625, 55.00000000000000000, -24.99999999999999645 ) ) ;
#7772=CARTESIAN_POINT ( 'NONE',  ( -74.37500000000000000, 30.00000000000000355, 4.592425496802573578E-15 ) ) ;
#7773=CARTESIAN_POINT ( 'NONE',  ( -75.00000000000000000, 40.74342228783053343, -21.53420582633694025 ) ) ;
#7788=CARTESIAN_POINT ( 'NONE',  ( -74.00000000204840944, 44.30836144126053000, 25.81189881250000795 ) ) ;
#7795=CARTESIAN_POINT ( 'NONE',  ( -77.18750000204838102, 44.30836144126052289, 25.81189881250000795 ) ) ;
#7797=DIRECTION ( 'NONE',  ( -1.000000000000000000, 0.000000000000000000, 0.000000000000000000 ) ) ;
#7807=CARTESIAN_POINT ( 'NONE',  ( -77.46875000000005684, 30.00000000000010303, 10.35533905932735443 ) ) ;
#7809=CIRCLE ( 'NONE', #8965, 25.00000000000000355 ) ;
#7829=CARTESIAN_POINT ( 'NONE',  ( -76.43750000409679046, 37.32233047033631124, 17.67766952966369232 ) ) ;
#7833=CARTESIAN_POINT ( 'NONE',  ( -72.40625000000000000, 65.35533905932737753, -24.99999999999999645 ) ) ;
#7848=CARTESIAN_POINT ( 'NONE',  ( -73.53125000204839523, 36.74823131438024859, -18.25176868561973720 ) ) ;
#7849=ORIENTED_EDGE ( 'NONE', *, *, #7125, .T. ) ;
#7852=EDGE_LOOP ( 'NONE', ( #10432, #1944, #2715, #225, #4477 ) ) ;
#7857=ADVANCED_BREP_SHAPE_REPRESENTATION ( '', ( #912, #4738 ), #3395 ) ;
#7870=CARTESIAN_POINT ( 'NONE',  ( -77.37500000000005684, 30.00000000000009592, 4.592425496802557801E-15 ) ) ;
#7878=CARTESIAN_POINT ( 'NONE',  ( -78.59375000204839523, 55.00000000000000000, 25.81189881249999729 ) ) ;
#7894=CARTESIAN_POINT ( 'NONE',  ( -78.59375000204839523, 36.74823131438026280, 18.25176868561974786 ) ) ;
#7908=CARTESIAN_POINT ( 'NONE',  ( -72.40625000204839523, 36.74823131438026280, 18.25176868561974786 ) ) ;
#7909=ORIENTED_EDGE ( 'NONE', *, *, #4193, .F. ) ;
#7914=ORIENTED_EDGE ( 'NONE', *, *, #8165, .T. ) ;
#7915=CARTESIAN_POINT ( 'NONE',  ( -77.75000000204839523, 80.81189881250000440, -10.69163855873948954 ) ) ;
#7924=ORIENTED_EDGE ( 'NONE', *, *, #10606, .T. ) ;
#7934=CARTESIAN_POINT ( 'NONE',  ( -75.31250000204839523, 29.18810118750000981, 10.69163855873950020 ) ) ;
#7949=CARTESIAN_POINT ( 'NONE',  ( -72.21875000000001421, 80.00000000000001421, -10.35533905932737753 ) ) ;
#7951=SHAPE_REPRESENTATION_RELATIONSHIP ( 'NONE' , 'NONE' ,  #6185, #7857 ) ;
#7956=ORIENTED_EDGE ( 'NONE', *, *, #1274, .F. ) ;
#7961=CARTESIAN_POINT ( 'NONE',  ( -71.84375000204838102, 55.00000000000000000, -25.81189881249999729 ) ) ;
#7969=CARTESIAN_POINT ( 'NONE',  ( -75.59375000204839523, 36.74823131438026280, 18.25176868561974786 ) ) ;
#7983=CARTESIAN_POINT ( 'NONE',  ( -77.18750000000007105, 37.32233047033638229, -17.67766952966361771 ) ) ;
#7988=CARTESIAN_POINT ( 'NONE',  ( -74.56250000204839523, 80.81189881250001861, -10.69163855873949132 ) ) ;
#7989=EDGE_CURVE ( 'NONE', #10082, #9652, #8774, .T. ) ;
#7997=CARTESIAN_POINT ( 'NONE',  ( -75.00000000000002842, 29.64870206142003539, -2.722520311965037632 ) ) ;
#7999=CARTESIAN_POINT ( 'NONE',  ( -75.12500000409677625, 55.00000000000000000, 24.99999999999999645 ) ) ;
#8009=CARTESIAN_POINT ( 'NONE',  ( -77.93750000204838102, 65.69163855873948421, -25.81189881250000440 ) ) ;
#8011=DIRECTION ( 'NONE',  ( 0.000000000000000000, 0.000000000000000000, 1.000000000000000000 ) ) ;
#8013=CARTESIAN_POINT ( 'NONE',  ( -79.90625000000001421, 65.35533905932736332, -24.99999999999996803 ) ) ;
#8021=CARTESIAN_POINT ( 'NONE',  ( -74.18750000204839523, 65.69163855873949842, 25.81189881250000440 ) ) ;
#8029=CARTESIAN_POINT ( 'NONE',  ( -75.96875000204839523, 73.25176868561975141, 18.25176868561974075 ) ) ;
#8030=AXIS2_PLACEMENT_3D ( 'NONE', #2134, #8491, #1416 ) ;
#8049=CARTESIAN_POINT ( 'NONE',  ( -76.71875000204839523, 29.18810118750000271, 4.741568889096522788E-15 ) ) ;
#8053=CARTESIAN_POINT ( 'NONE',  ( -76.90625000409677625, 80.00000000000001421, 10.35533905932737397 ) ) ;
#8072=CARTESIAN_POINT ( 'NONE',  ( -71.75000000204838102, 80.81189881250001861, -10.69163855873949132 ) ) ;
#8099=CARTESIAN_POINT ( 'NONE',  ( -76.15625000204838102, 80.81189881250000440, -1.580522963032174394E-15 ) ) ;
#8110=CARTESIAN_POINT ( 'NONE',  ( -76.06250000409679046, 37.32233047033631124, -17.67766952966368166 ) ) ;
#8111=CARTESIAN_POINT ( 'NONE',  ( -76.43750000204839523, 44.30836144126050158, -25.81189881249999374 ) ) ;
#8118=VECTOR ( 'NONE', #638, 1000.000000000000000 ) ;
#8124=CARTESIAN_POINT ( 'NONE',  ( -71.93750000204838102, 65.69163855873948421, -25.81189881250000440 ) ) ;
#8133=CARTESIAN_POINT ( 'NONE',  ( -80.00000000000000000, 55.00000000000000000, 0.000000000000000000 ) ) ;
#8150=CARTESIAN_POINT ( 'NONE',  ( -79.34375000204839523, 73.25176868561975141, -18.25176868561974430 ) ) ;
#8157=CARTESIAN_POINT ( 'NONE',  ( -75.78125000204839523, 73.25176868561975141, 18.25176868561974075 ) ) ;
#8164=CARTESIAN_POINT ( 'NONE',  ( -75.40625000409677625, 80.00000000000001421, 10.35533905932737397 ) ) ;
#8165=EDGE_CURVE ( 'NONE', #10833, #1407, #9136, .T. ) ;
#8167=CARTESIAN_POINT ( 'NONE',  ( -80.00000000000000000, 55.00000000000000000, 0.000000000000000000 ) ) ;
#8183=CARTESIAN_POINT ( 'NONE',  ( -74.37500000204838102, 65.69163855873949842, 25.81189881250000440 ) ) ;
#8197=VERTEX_POINT ( 'NONE', #4461 ) ;
#8208=CARTESIAN_POINT ( 'NONE',  ( -76.90625000204838102, 29.18810118750000271, 4.741568889096522788E-15 ) ) ;
#8217=CARTESIAN_POINT ( 'NONE',  ( -77.00000000204839523, 44.30836144126052289, 25.81189881250000795 ) ) ;
#8220=CIRCLE ( 'NONE', #9357, 29.00000000000000355 ) ;
#8225=CARTESIAN_POINT ( 'NONE',  ( -78.21875000409679046, 65.35533905932737753, 24.99999999999999645 ) ) ;
#8239=CARTESIAN_POINT ( 'NONE',  ( -75.40625000204838102, 29.18810118750000271, 4.741568889096522788E-15 ) ) ;
#8246=EDGE_LOOP ( 'NONE', ( #6667, #7323, #2676, #5787, #6060 ) ) ;
#8248=AXIS2_PLACEMENT_3D ( 'NONE', #5886, #3961, #3063 ) ;
#8266=EDGE_CURVE ( 'NONE', #8197, #10439, #9784, .T. ) ;
#8268=CARTESIAN_POINT ( 'NONE',  ( -77.00000000204838102, 29.18810118750000981, 10.69163855873950020 ) ) ;
#8274=CARTESIAN_POINT ( 'NONE',  ( -76.71875000204839523, 29.18810118750000271, 4.741568889096522788E-15 ) ) ;
#8279=CARTESIAN_POINT ( 'NONE',  ( -71.65625000204839523, 73.25176868561975141, -18.25176868561974430 ) ) ;
#8295=CARTESIAN_POINT ( 'NONE',  ( -75.68750000204838102, 44.30836144126053000, 25.81189881250000795 ) ) ;
#8308=ORIENTED_EDGE ( 'NONE', *, *, #7559, .F. ) ;
#8328=CARTESIAN_POINT ( 'NONE',  ( -79.15625000204839523, 73.25176868561975141, -18.25176868561974430 ) ) ;
#8329=CARTESIAN_POINT ( 'NONE',  ( -74.99999999999998579, 79.77762491170771852, 4.737166167340707723 ) ) ;
#8334=CARTESIAN_POINT ( 'NONE',  ( -71.34302368722833876, 77.35376350879521112, 12.90594348738575903 ) ) ;
#8335=DIRECTION ( 'NONE',  ( -1.000000000000000000, 0.000000000000000000, 0.000000000000000000 ) ) ;
#8343=CARTESIAN_POINT ( 'NONE',  ( -79.71875000000000000, 79.99999999999998579, -10.35533905932736332 ) ) ;
#8358=EDGE_LOOP ( 'NONE', ( #11222, #7909, #10484, #9164, #3130, #7914, #2287, #4560, #8832 ) ) ;
#8361=CARTESIAN_POINT ( 'NONE',  ( -78.50000000000000000, 55.00000000000000000, -24.99999999999999645 ) ) ;
#8370=CARTESIAN_POINT ( 'NONE',  ( -75.50000000409677625, 80.00000000000000000, -1.530808498934191324E-15 ) ) ;
#8372=( BOUNDED_CURVE ( )  B_SPLINE_CURVE ( 2, ( #6041, #3994, #9677, #10335, #451, #5805, #7654, #9439, #1228 ),
 .UNSPECIFIED., .F., .T. ) 
 B_SPLINE_CURVE_WITH_KNOTS ( ( 3, 2, 2, 2, 3 ),
 ( 0.07919667986333785159, 0.09899957127346223351, 0.1188024626835866154, 0.1386053540937109974, 0.1584082455038353654 ),
 .UNSPECIFIED. ) 
 CURVE ( )  GEOMETRIC_REPRESENTATION_ITEM ( )  RATIONAL_B_SPLINE_CURVE ( ( 0.9999999999999998890, 0.9238795325112866275, 0.9999999999999998890, 0.9238795325112866275, 0.9999999999999998890, 0.9238795325112866275, 0.9999999999999998890, 0.9238795325113071666, 0.9999999999999793499 ) ) 
 REPRESENTATION_ITEM ( '' )  );
#8373=CARTESIAN_POINT ( 'NONE',  ( -79.43750000000001421, 72.67766952966368876, 17.67766952966368521 ) ) ;
#8387=CARTESIAN_POINT ( 'NONE',  ( -78.78125000204839523, 73.25176868561975141, 18.25176868561974075 ) ) ;
#8389=VERTEX_POINT ( 'NONE', #6909 ) ;
#8399=CARTESIAN_POINT ( 'NONE',  ( -76.25000000409677625, 30.00000000000000355, 4.592425496802573578E-15 ) ) ;
#8410=EDGE_CURVE ( 'NONE', #5247, #10943, #7088, .T. ) ;
#8423=DIRECTION ( 'NONE',  ( -1.000000000000000000, 0.000000000000000000, 0.000000000000000000 ) ) ;
#8433=CARTESIAN_POINT ( 'NONE',  ( -75.50000000000000000, 55.00000000000000000, -24.99999999999999645 ) ) ;
#8444=VERTEX_POINT ( 'NONE', #480 ) ;
#8451=CARTESIAN_POINT ( 'NONE',  ( -72.21875000204838102, 36.74823131438024859, -18.25176868561973720 ) ) ;
#8452=ORIENTED_EDGE ( 'NONE', *, *, #7989, .T. ) ;
#8460=CARTESIAN_POINT ( 'NONE',  ( -79.06250000204839523, 80.81189881250000440, 10.69163855873948243 ) ) ;
#8461=CARTESIAN_POINT ( 'NONE',  ( -74.99999999999998579, 76.80627241285399975, -13.27287850887629084 ) ) ;
#8475=VERTEX_POINT ( 'NONE', #5226 ) ;
#8484=B_SPLINE_CURVE_WITH_KNOTS ( 'NONE', 1,
 ( #1104, #2915 ),
 .UNSPECIFIED., .F., .F.,
 ( 2, 2 ),
 ( 0.000000000000000000, 1.000000000000000000 ),
 .UNSPECIFIED. ) ;
#8491=DIRECTION ( 'NONE',  ( -1.000000000000000000, 0.000000000000000000, 0.000000000000000000 ) ) ;
#8496=CARTESIAN_POINT ( 'NONE',  ( -78.87500000000000000, 30.00000000000000355, 4.592425496802573578E-15 ) ) ;
#8508=CARTESIAN_POINT ( 'NONE',  ( -77.75000000204839523, 65.69163855873948421, -25.81189881250000440 ) ) ;
#8516=CARTESIAN_POINT ( 'NONE',  ( -74.99999999999998579, 78.53260953835976466, -9.507204588591818606 ) ) ;
#8521=CARTESIAN_POINT ( 'NONE',  ( -74.93750000409677625, 37.32233047033631124, 17.67766952966369232 ) ) ;
#8554=CARTESIAN_POINT ( 'NONE',  ( -75.68750000000000000, 37.32233047033631124, -17.67766952966368166 ) ) ;
#8555=CARTESIAN_POINT ( 'NONE',  ( -75.00000000000001421, 58.46699551781524917, -25.57799957749213604 ) ) ;
#8568=CARTESIAN_POINT ( 'NONE',  ( -77.09375000204839523, 55.00000000000000000, 25.81189881249999729 ) ) ;
#8572=CARTESIAN_POINT ( 'NONE',  ( -75.68750000000005684, 37.32233047033638940, -17.67766952966360705 ) ) ;
#8586=CARTESIAN_POINT ( 'NONE',  ( -71.09375000409677625, 80.00000000000001421, -10.35533905932737753 ) ) ;
#8618=CARTESIAN_POINT ( 'NONE',  ( -76.43750000000000000, 72.67766952966368876, 17.67766952966368521 ) ) ;
#8629=CARTESIAN_POINT ( 'NONE',  ( -73.34375000204839523, 73.25176868561975141, -18.25176868561974430 ) ) ;
#8636=PLANE ( 'NONE',  #8248 ) ;
#8637=FACE_BOUND ( 'NONE', #10004, .T. ) ;
#8644=CARTESIAN_POINT ( 'NONE',  ( -75.00000000000000000, 55.00000000000000000, 0.000000000000000000 ) ) ;
#8672=DIRECTION ( 'NONE',  ( -1.000000000000000000, 0.000000000000000000, 0.000000000000000000 ) ) ;
#8674=CARTESIAN_POINT ( 'NONE',  ( -73.34375000000001421, 65.35533905932737753, 24.99999999999999645 ) ) ;
#8677=FACE_OUTER_BOUND ( 'NONE', #6092, .T. ) ;
#8686=CARTESIAN_POINT ( 'NONE',  ( -73.90625000204839523, 36.74823131438026280, 18.25176868561974786 ) ) ;
#8700=ADVANCED_FACE ( 'NONE', ( #1988 ), #9358, .F. ) ;
#8710=ORIENTED_EDGE ( 'NONE', *, *, #4053, .F. ) ;
#8723=CARTESIAN_POINT ( 'NONE',  ( -76.34375000409679046, 30.00000000000001421, 10.35533905932739174 ) ) ;
#8728=CARTESIAN_POINT ( 'NONE',  ( -78.68750000204838102, 44.30836144126053000, 25.81189881250000795 ) ) ;
#8729=CARTESIAN_POINT ( 'NONE',  ( -74.99999999999997158, 47.61856851181366324, -24.74822985635785599 ) ) ;
#8742=CARTESIAN_POINT ( 'NONE',  ( -74.37500000204838102, 80.81189881250001861, 10.69163855873948599 ) ) ;
#8746=CARTESIAN_POINT ( 'NONE',  ( -75.96875000000005684, 30.00000000000011013, 10.35533905932735088 ) ) ;
#8763=CARTESIAN_POINT ( 'NONE',  ( -83.00000000000000000, 55.00000000000000000, 0.000000000000000000 ) ) ;
#8770=CARTESIAN_POINT ( 'NONE',  ( -79.06250000204840944, 80.81189881250001861, -10.69163855873949132 ) ) ;
#8774=LINE ( 'NONE', #3319, #5589 ) ;
#8776=CARTESIAN_POINT ( 'NONE',  ( -75.00000000000000000, 31.79283308196307445, 9.999956478894377554 ) ) ;
#8787=CARTESIAN_POINT ( 'NONE',  ( -73.62500000000000000, 80.00000000000000000, -1.530808498934191324E-15 ) ) ;
#8803=CARTESIAN_POINT ( 'NONE',  ( -72.87500000204840944, 80.81189881250001861, 10.69163855873948599 ) ) ;
#8809=CARTESIAN_POINT ( 'NONE',  ( -75.00000000000001421, 58.46699551781524917, -25.57799957749213604 ) ) ;
#8814=DIRECTION ( 'NONE',  ( 0.000000000000000000, 0.000000000000000000, 1.000000000000000000 ) ) ;
#8827=CARTESIAN_POINT ( 'NONE',  ( -78.87500000409677625, 55.00000000000000000, -24.99999999999999645 ) ) ;
#8830=VECTOR ( 'NONE', #11132, 1000.000000000000000 ) ;
#8832=ORIENTED_EDGE ( 'NONE', *, *, #11645, .T. ) ;
#8833=CARTESIAN_POINT ( 'NONE',  ( -76.34375000204839523, 55.00000000000000000, -25.81189881249999729 ) ) ;
#8849=CARTESIAN_POINT ( 'NONE',  ( -74.56250000000000000, 37.32233047033631124, 17.67766952966369232 ) ) ;
#8862=CARTESIAN_POINT ( 'NONE',  ( -73.06250000204840944, 80.81189881250001861, -10.69163855873949132 ) ) ;
#8869=CARTESIAN_POINT ( 'NONE',  ( -75.78125000204838102, 55.00000000000000000, 25.81189881249999729 ) ) ;
#8886=VERTEX_POINT ( 'NONE', #1336 ) ;
#8888=CARTESIAN_POINT ( 'NONE',  ( -76.90625000204839523, 36.74823131438026280, 18.25176868561974786 ) ) ;
#8893=CARTESIAN_POINT ( 'NONE',  ( -75.00000000000000000, 30.98212383677083892, -8.811831842167247686 ) ) ;
#8903=CARTESIAN_POINT ( 'NONE',  ( -72.68750000000000000, 37.32233047033631124, -17.67766952966368166 ) ) ;
#8905=PRESENTATION_STYLE_ASSIGNMENT (( #5044 ) ) ;
#8915=CARTESIAN_POINT ( 'NONE',  ( -71.75000000204840944, 65.69163855873948421, -25.81189881250000440 ) ) ;
#8950=CARTESIAN_POINT ( 'NONE',  ( -78.68750000204839523, 65.69163855873949842, 25.81189881250000440 ) ) ;
#8957=CARTESIAN_POINT ( 'NONE',  ( -74.99999999999995737, 40.75327862118771804, 20.61280595097384349 ) ) ;
#8965=AXIS2_PLACEMENT_3D ( 'NONE', #4134, #7797, #8814 ) ;
#8967=CARTESIAN_POINT ( 'NONE',  ( -72.96875000204838102, 73.25176868561975141, 18.25176868561974075 ) ) ;
#8973=EDGE_LOOP ( 'NONE', ( #559, #11783 ) ) ;
#8994=CARTESIAN_POINT ( 'NONE',  ( -74.93750000204839523, 65.69163855873948421, -25.81189881250000440 ) ) ;
#9001=CARTESIAN_POINT ( 'NONE',  ( -78.31250000204839523, 29.18810118750000981, 10.69163855873950020 ) ) ;
#9006=CARTESIAN_POINT ( 'NONE',  ( -73.53125000204839523, 36.74823131438024859, -18.25176868561973720 ) ) ;
#9024=CARTESIAN_POINT ( 'NONE',  ( -73.81250000204839523, 29.18810118750000626, -10.69163855873949309 ) ) ;
#9027=EDGE_CURVE ( 'NONE', #11066, #8197, #1744, .T. ) ;
#9038=DIRECTION ( 'NONE',  ( -1.000000000000000000, 0.000000000000000000, 0.000000000000000000 ) ) ;
#9049=CARTESIAN_POINT ( 'NONE',  ( -79.53125000204838102, 55.00000000000000000, -25.81189881249999729 ) ) ;
#9055=CARTESIAN_POINT ( 'NONE',  ( -78.40625000204839523, 36.74823131438026280, 18.25176868561974786 ) ) ;
#9061=CARTESIAN_POINT ( 'NONE',  ( -75.68750000409677625, 72.67766952966368876, -17.67766952966368876 ) ) ;
#9077=CARTESIAN_POINT ( 'NONE',  ( -73.25000000204838102, 80.81189881250001861, -10.69163855873949132 ) ) ;
#9094=STYLED_ITEM('',(#11874),#912);
#9097=LINE ( 'NONE', #3529, #693 ) ;
#9103=CARTESIAN_POINT ( 'NONE',  ( -79.06250000204839523, 80.81189881250001861, 10.69163855873948599 ) ) ;
#9113=CARTESIAN_POINT ( 'NONE',  ( -79.43750000204838102, 55.00000000000000000, -25.81189881249999729 ) ) ;
#9116=CARTESIAN_POINT ( 'NONE',  ( -76.43750000409679046, 37.32233047033631124, 17.67766952966369232 ) ) ;
#9121=AXIS2_PLACEMENT_3D ( 'NONE', #7740, #9529, #475 ) ;
#9133=CARTESIAN_POINT ( 'NONE',  ( -76.34375000204839523, 73.25176868561975141, -18.25176868561974430 ) ) ;
#9136=( BOUNDED_CURVE ( )  B_SPLINE_CURVE ( 2, ( #9840, #9955, #2658, #10788, #7107, #8053, #11696, #3497, #728 ),
 .UNSPECIFIED., .F., .T. ) 
 B_SPLINE_CURVE_WITH_KNOTS ( ( 3, 2, 2, 2, 3 ),
 ( 0.1666666666666667962, 0.1875000000000001665, 0.2083333333333335369, 0.2291666666666668517, 0.2500000000000002220 ),
 .UNSPECIFIED. ) 
 CURVE ( )  GEOMETRIC_REPRESENTATION_ITEM ( )  RATIONAL_B_SPLINE_CURVE ( ( 0.9999999999999994449, 0.9238795325112872936, 1.000000000000000000, 0.9238795325112867385, 1.000000000000000000, 0.9238795325112867385, 1.000000000000000000, 0.9238795325112859613, 1.000000000000000888 ) ) 
 REPRESENTATION_ITEM ( '' )  );
#9161=CARTESIAN_POINT ( 'NONE',  ( -78.21875000204839523, 36.74823131438024859, -18.25176868561973720 ) ) ;
#9164=ORIENTED_EDGE ( 'NONE', *, *, #4012, .T. ) ;
#9169=LINE ( 'NONE', #953, #5196 ) ;
#9170=CARTESIAN_POINT ( 'NONE',  ( -75.00000000000002842, 79.21399255846120013, -7.542952894479948434 ) ) ;
#9171=DIRECTION ( 'NONE',  ( 0.000000000000000000, -0.000000000000000000, -1.000000000000000000 ) ) ;
#9176=CARTESIAN_POINT ( 'NONE',  ( -78.12500000409677625, 55.00000000000000000, 24.99999999999999645 ) ) ;
#9184=CARTESIAN_POINT ( 'NONE',  ( -76.25000000000000000, 55.00000000000000000, 24.99999999999999645 ) ) ;
#9188=ORIENTED_EDGE ( 'NONE', *, *, #307, .F. ) ;
#9189=CARTESIAN_POINT ( 'NONE',  ( -74.65625000204838102, 80.81189881250000440, -1.580522963032174394E-15 ) ) ;
#9215=ORIENTED_EDGE ( 'NONE', *, *, #11645, .F. ) ;
#9221=CARTESIAN_POINT ( 'NONE',  ( -75.12500000204838102, 44.30836144126050158, -25.81189881249999374 ) ) ;
#9233=CARTESIAN_POINT ( 'NONE',  ( -72.78125000204839523, 73.25176868561975141, 18.25176868561974075 ) ) ;
#9234=EDGE_CURVE ( 'NONE', #131, #9375, #763, .T. ) ;
#9255=FACE_OUTER_BOUND ( 'NONE', #1993, .T. ) ;
#9262=CARTESIAN_POINT ( 'NONE',  ( -77.84375000000001421, 65.35533905932737753, 24.99999999999999645 ) ) ;
#9274=CARTESIAN_POINT ( 'NONE',  ( -78.50000000204840944, 44.30836144126053000, 25.81189881250000795 ) ) ;
#9282=CARTESIAN_POINT ( 'NONE',  ( -75.00000000000000000, 78.32225602221440397, 9.188098902483863739 ) ) ;
#9287=CARTESIAN_POINT ( 'NONE',  ( -76.62500000409677625, 55.00000000000000000, 24.99999999999999645 ) ) ;
#9306=ADVANCED_FACE ( 'NONE', ( #2219, #8637 ), #418, .F. ) ;
#9325=CARTESIAN_POINT ( 'NONE',  ( -75.87500000000000000, 30.00000000000000355, 4.592425496802573578E-15 ) ) ;
#9338=CARTESIAN_POINT ( 'NONE',  ( -72.31250000204839523, 29.18810118750000626, -10.69163855873949309 ) ) ;
#9347=CARTESIAN_POINT ( 'NONE',  ( -75.00000000000000000, 79.90134559235561085, -4.530844741510550833 ) ) ;
#9351=CARTESIAN_POINT ( 'NONE',  ( -72.87500000409677625, 55.00000000000000000, -24.99999999999999645 ) ) ;
#9357=AXIS2_PLACEMENT_3D ( 'NONE', #5324, #2564, #1657 ) ;
#9358=CYLINDRICAL_SURFACE ( 'NONE', #4715, 25.00000000000000355 ) ;
#9364=CARTESIAN_POINT ( 'NONE',  ( -79.34375000204839523, 55.00000000000000000, -25.81189881249999729 ) ) ;
#9375=VERTEX_POINT ( 'NONE', #3236 ) ;
#9378=CARTESIAN_POINT ( 'NONE',  ( -77.93750000409679046, 37.32233047033631124, 17.67766952966369232 ) ) ;
#9381=CARTESIAN_POINT ( 'NONE',  ( -75.31250000409677625, 72.67766952966368876, 17.67766952966368521 ) ) ;
#9384=CARTESIAN_POINT ( 'NONE',  ( -77.65625000000001421, 44.64466094067262958, 25.00000000000001066 ) ) ;
#9385=CARTESIAN_POINT ( 'NONE',  ( -74.99999999999997158, 57.62508896066697872, -25.69211664326230604 ) ) ;
#9399=CARTESIAN_POINT ( 'NONE',  ( -74.18750000204838102, 44.30836144126053000, 25.81189881250000795 ) ) ;
#9408=CARTESIAN_POINT ( 'NONE',  ( -75.00000000000001421, 75.69461608703821298, -15.00647013622189618 ) ) ;
#9413=CARTESIAN_POINT ( 'NONE',  ( -74.56250000409677625, 37.32233047033631124, -17.67766952966368166 ) ) ;
#9420=VERTEX_POINT ( 'NONE', #5104 ) ;
#9433=EDGE_CURVE ( 'NONE', #2377, #1407, #9097, .T. ) ;
#9435=CARTESIAN_POINT ( 'NONE',  ( -78.21875000000004263, 79.99999999999992895, -10.35533905932734910 ) ) ;
#9439=CARTESIAN_POINT ( 'NONE',  ( -78.59375000000001421, 44.64466094067047663, -24.99999999999782219 ) ) ;
#9442=CARTESIAN_POINT ( 'NONE',  ( -75.12500000000007105, 79.99999999999990052, -1.530808498934185013E-15 ) ) ;
#9451=CYLINDRICAL_SURFACE ( 'NONE', #125, 25.00000000000000355 ) ;
#9460=CARTESIAN_POINT ( 'NONE',  ( -72.40625000204838102, 29.18810118750000271, 4.741568889096522788E-15 ) ) ;
#9474=CARTESIAN_POINT ( 'NONE',  ( -74.84375000409679046, 30.00000000000001421, 10.35533905932739174 ) ) ;
#9505=CARTESIAN_POINT ( 'NONE',  ( -79.15625000000000000, 44.64466094067262958, 25.00000000000001066 ) ) ;
#9520=CARTESIAN_POINT ( 'NONE',  ( -74.65625000204838102, 80.81189881250000440, -1.580522963032174394E-15 ) ) ;
#9525=SURFACE_SIDE_STYLE ('',( #2553 ) ) ;
#9529=DIRECTION ( 'NONE',  ( -1.000000000000000000, 0.000000000000000000, 0.000000000000000000 ) ) ;
#9535=CARTESIAN_POINT ( 'NONE',  ( -71.75000000409677625, 30.00000000000000355, 4.592425496802573578E-15 ) ) ;
#9566=FACE_OUTER_BOUND ( 'NONE', #4579, .T. ) ;
#9568=CARTESIAN_POINT ( 'NONE',  ( -74.46875000000000000, 30.00000000000001421, 10.35533905932739174 ) ) ;
#9581=ORIENTED_EDGE ( 'NONE', *, *, #6453, .F. ) ;
#9587=CIRCLE ( 'NONE', #401, 29.00000000000000355 ) ;
#9600=( BOUNDED_CURVE ( )  B_SPLINE_CURVE ( 2, ( #3038, #2358, #6525, #10277, #9442, #6029, #1231 ),
 .UNSPECIFIED., .F., .T. ) 
 B_SPLINE_CURVE_WITH_KNOTS ( ( 3, 2, 2, 3 ),
 ( 0.4753074076739236542, 0.4951195077574221948, 0.5149316078409206243, 0.5280270264772872757 ),
 .UNSPECIFIED. ) 
 CURVE ( )  GEOMETRIC_REPRESENTATION_ITEM ( )  RATIONAL_B_SPLINE_CURVE ( ( 0.9999999999998887557, 0.9238795325113978718, 0.9999999999999998890, 0.9238795325112867385, 0.9999999999999998890, 0.9496858291468608382, 0.9658850645340137930 ) ) 
 REPRESENTATION_ITEM ( '' )  );
#9623=CARTESIAN_POINT ( 'NONE',  ( -79.43750000204838102, 55.00000000000000000, -25.81189881249999729 ) ) ;
#9625=CARTESIAN_POINT ( 'NONE',  ( -72.59375000000000000, 44.64466094067260826, -24.99999999999998934 ) ) ;
#9636=CARTESIAN_POINT ( 'NONE',  ( -75.68750000204839523, 65.69163855873949842, 25.81189881250000440 ) ) ;
#9652=VERTEX_POINT ( 'NONE', #7548 ) ;
#9661=CARTESIAN_POINT ( 'NONE',  ( -76.25000000204838102, 65.69163855873948421, -25.81189881250000440 ) ) ;
#9663=MECHANICAL_DESIGN_GEOMETRIC_PRESENTATION_REPRESENTATION('',(#9094),#478);
#9668=CARTESIAN_POINT ( 'NONE',  ( -75.00000000000000000, 31.54307055854626540, -10.27649223703322612 ) ) ;
#9677=CARTESIAN_POINT ( 'NONE',  ( -79.06250000000002842, 37.32233047033633966, 17.67766952966367100 ) ) ;
#9682=CARTESIAN_POINT ( 'NONE',  ( -74.09375000000000000, 44.64466094067260826, -24.99999999999998934 ) ) ;
#9694=CARTESIAN_POINT ( 'NONE',  ( -75.40625000204839523, 36.74823131438026280, 18.25176868561974786 ) ) ;
#9702=CARTESIAN_POINT ( 'NONE',  ( -75.00000000000000000, 76.68791387293471473, 12.43520775219157315 ) ) ;
#9711=ADVANCED_FACE ( 'NONE', ( #1237 ), #515, .T. ) ;
#9718=CARTESIAN_POINT ( 'NONE',  ( -77.00000000204838102, 44.30836144126053000, 25.81189881250000795 ) ) ;
#9734=CARTESIAN_POINT ( 'NONE',  ( -72.50000000000000000, 55.00000000000000000, -24.99999999999999645 ) ) ;
#9748=CARTESIAN_POINT ( 'NONE',  ( -73.81250000204839523, 29.18810118750000981, 10.69163855873950020 ) ) ;
#9756=CARTESIAN_POINT ( 'NONE',  ( -77.56250000204838102, 80.81189881250000440, 10.69163855873948243 ) ) ;
#9776=AXIS2_PLACEMENT_3D ( 'NONE', #8763, #5171, #11439 ) ;
#9779=CARTESIAN_POINT ( 'NONE',  ( -75.59375000204839523, 55.00000000000000000, 25.81189881249999729 ) ) ;
#9784=CIRCLE ( 'NONE', #3292, 20.00000000000000355 ) ;
#9785=CARTESIAN_POINT ( 'NONE',  ( -75.00000000000001421, 31.01194267615668920, 8.057582179793557842 ) ) ;
#9795=CARTESIAN_POINT ( 'NONE',  ( -73.53125000000000000, 80.00000000000001421, 10.35533905932737397 ) ) ;
#9798=CYLINDRICAL_SURFACE ( 'NONE', #7453, 25.00000000000000355 ) ;
#9805=FACE_OUTER_BOUND ( 'NONE', #7852, .T. ) ;
#9806=CARTESIAN_POINT ( 'NONE',  ( -71.34302368722833876, 77.35376350879521112, 12.90594348738575903 ) ) ;
#9827=ORIENTED_EDGE ( 'NONE', *, *, #7718, .T. ) ;
#9832=VECTOR ( 'NONE', #3114, 1000.000000000000000 ) ;
#9838=CARTESIAN_POINT ( 'NONE',  ( -77.09375000204839523, 55.00000000000000000, 25.81189881249999729 ) ) ;
#9840=CARTESIAN_POINT ( 'NONE',  ( -77.37500000409677625, 55.00000000000000000, -24.99999999999999645 ) ) ;
#9852=CARTESIAN_POINT ( 'NONE',  ( -73.62500000204839523, 44.30836144126050158, -25.81189881249999374 ) ) ;
#9864=VERTEX_POINT ( 'NONE', #402 ) ;
#9886=CARTESIAN_POINT ( 'NONE',  ( -76.34375000204839523, 55.00000000000000000, -25.81189881249999729 ) ) ;
#9894=ADVANCED_FACE ( 'NONE', ( #8677 ), #9451, .F. ) ;
#9895=CARTESIAN_POINT ( 'NONE',  ( -73.90625000204839523, 36.74823131438026280, 18.25176868561974786 ) ) ;
#9902=CARTESIAN_POINT ( 'NONE',  ( -75.00000000000001421, 29.78398716281686021, 3.536572121053506823 ) ) ;
#9911=CARTESIAN_POINT ( 'NONE',  ( -76.15625000204838102, 80.81189881250000440, -1.580522963032174394E-15 ) ) ;
#9915=DIRECTION ( 'NONE',  ( 0.000000000000000000, 0.000000000000000000, 1.000000000000000000 ) ) ;
#9922=DIRECTION ( 'NONE',  ( -1.000000000000000000, 0.000000000000000000, 0.000000000000000000 ) ) ;
#9939=FACE_OUTER_BOUND ( 'NONE', #3487, .T. ) ;
#9947=CARTESIAN_POINT ( 'NONE',  ( -78.50000000204842365, 44.30836144126052289, 25.81189881250000795 ) ) ;
#9952=CARTESIAN_POINT ( 'NONE',  ( -78.78125000409679046, 65.35533905932737753, -24.99999999999999645 ) ) ;
#9955=CARTESIAN_POINT ( 'NONE',  ( -77.28125000409677625, 65.35533905932743437, -24.99999999999994671 ) ) ;
#9968=EDGE_CURVE ( 'NONE', #10943, #8444, #7394, .T. ) ;
#9969=CARTESIAN_POINT ( 'NONE',  ( -73.71875000204839523, 36.74823131438024859, -18.25176868561973720 ) ) ;
#9971=( BOUNDED_CURVE ( )  B_SPLINE_CURVE ( 2, ( #1134, #2096, #417, #4079, #4802, #8460, #10182, #238, #5829, #5769, #7679, #11315, #3123, #6788, #2218, #7738, #6184, #10589, #532, #7915, #2390, #9756, #4377, #11544, #2456, #7795, #4256, #6122, #3348, #6964, #7020, #4311, #1498, #3410, #11485, #10643, #6066, #6904, #8029, #649, #8869, #5221, #7969, #4195, #5157, #1555, #3295, #11605, #705, #7083, #3178 ),
 .UNSPECIFIED., .F., .T. ) 
 B_SPLINE_CURVE_WITH_KNOTS ( ( 3, 2, 2, 2, 2, 2, 2, 2, 2, 2, 2, 2, 2, 2, 2, 2, 2, 2, 2, 2, 2, 2, 2, 2, 2, 3 ),
 ( 0.000000000000000000, 0.02083333333333333218, 0.04166666666666666435, 0.06250000000000000000, 0.08333333333333332871, 0.1041666666666666713, 0.1250000000000000000, 0.1458333333333333426, 0.1666666666666666574, 0.1875000000000000000, 0.2083333333333333426, 0.2291666666666666574, 0.2500000000000000000, 0.2708333333333333148, 0.2916666666666666852, 0.3125000000000000000, 0.3333333333333333148, 0.3541666666666666852, 0.3750000000000000000, 0.3958333333333333148, 0.4166666666666666852, 0.4375000000000000000, 0.4583333333333333148, 0.4791666666666666852, 0.5000000000000000000, 0.5036241432350977432 ),
 .UNSPECIFIED. ) 
 CURVE ( )  GEOMETRIC_REPRESENTATION_ITEM ( )  RATIONAL_B_SPLINE_CURVE ( ( 1.000000000000000000, 0.9238795325112867385, 1.000000000000000000, 0.9238795325112867385, 1.000000000000000000, 0.9238795325112867385, 1.000000000000000000, 0.9238795325112867385, 1.000000000000000000, 0.9238795325112867385, 1.000000000000000000, 0.9238795325112867385, 1.000000000000000000, 0.9238795325112867385, 1.000000000000000000, 0.9238795325112867385, 1.000000000000000000, 0.9238795325112867385, 1.000000000000000000, 0.9238795325112867385, 1.000000000000000000, 0.9238795325112867385, 1.000000000000000000, 0.9238795325112867385, 1.000000000000000000, 0.9238795325112867385, 1.000000000000000000, 0.9238795325112867385, 1.000000000000000000, 0.9238795325112867385, 1.000000000000000000, 0.9238795325112867385, 1.000000000000000000, 0.9238795325112867385, 1.000000000000000000, 0.9238795325112867385, 1.000000000000000000, 0.9238795325112867385, 1.000000000000000000, 0.9238795325112867385, 1.000000000000000000, 0.9238795325112867385, 1.000000000000000000, 0.9238795325112867385, 1.000000000000000000, 0.9238795325112867385, 1.000000000000000000, 0.9238795325112867385, 1.000000000000000000, 0.9867581690895185220, 0.9781234062028318910 ) ) 
 REPRESENTATION_ITEM ( '' )  );
#9979=LINE ( 'NONE', #10986, #11664 ) ;
#9994=CARTESIAN_POINT ( 'NONE',  ( -78.12500000204838102, 44.30836144126050158, -25.81189881249999374 ) ) ;
#10000=CARTESIAN_POINT ( 'NONE',  ( -75.01598058408755776, 37.97957837300059225, -19.48311574424008086 ) ) ;
#10004=EDGE_LOOP ( 'NONE', ( #5027, #2868, #6336, #7924, #6209 ) ) ;
#10005=( LENGTH_UNIT ( ) NAMED_UNIT ( * ) SI_UNIT ( .MILLI., .METRE. ) );
#10006=CARTESIAN_POINT ( 'NONE',  ( -76.81250000409679046, 72.67766952966368876, 17.67766952966368521 ) ) ;
#10021=CARTESIAN_POINT ( 'NONE',  ( -74.75000000204839523, 80.81189881250001861, -10.69163855873949132 ) ) ;
#10048=CARTESIAN_POINT ( 'NONE',  ( -75.87500000204839523, 65.69163855873949842, 25.81189881250000440 ) ) ;
#10057=CARTESIAN_POINT ( 'NONE',  ( -74.99999999999997158, 67.69301918158085130, -22.29621844334601377 ) ) ;
#10063=CARTESIAN_POINT ( 'NONE',  ( -73.15625000204839523, 73.25176868561975141, -18.25176868561974430 ) ) ;
#10070=ORIENTED_EDGE ( 'NONE', *, *, #6469, .T. ) ;
#10076=AXIS2_PLACEMENT_3D ( 'NONE', #4454, #4506, #958 ) ;
#10078=CARTESIAN_POINT ( 'NONE',  ( -73.15625000204838102, 80.81189881250000440, -1.580522963032174394E-15 ) ) ;
#10082=VERTEX_POINT ( 'NONE', #4694 ) ;
#10107=CARTESIAN_POINT ( 'NONE',  ( -75.31250000204839523, 29.18810118750000626, -10.69163855873949309 ) ) ;
#10108=ORIENTED_EDGE ( 'NONE', *, *, #8410, .F. ) ;
#10116=CARTESIAN_POINT ( 'NONE',  ( -75.40625000204839523, 36.74823131438026280, 18.25176868561974786 ) ) ;
#10117=CARTESIAN_POINT ( 'NONE',  ( -74.99999999999998579, 68.14082849008082121, -22.02527069007740934 ) ) ;
#10122=CARTESIAN_POINT ( 'NONE',  ( -77.75000000409677625, 30.00000000000000355, 4.592425496802573578E-15 ) ) ;
#10146=CARTESIAN_POINT ( 'NONE',  ( -77.75000000000000000, 55.00000000000000000, 24.99999999999999645 ) ) ;
#10173=CARTESIAN_POINT ( 'NONE',  ( -76.34375000204839523, 73.25176868561975141, -18.25176868561974430 ) ) ;
#10182=CARTESIAN_POINT ( 'NONE',  ( -78.96875000204839523, 73.25176868561975141, 18.25176868561974075 ) ) ;
#10183=CARTESIAN_POINT ( 'NONE',  ( -75.00000000000000000, 78.87322666461865595, 7.729222434168494971 ) ) ;
#10190=CARTESIAN_POINT ( 'NONE',  ( -77.28125000409677625, 65.35533905932737753, -24.99999999999999645 ) ) ;
#10207=ORIENTED_EDGE ( 'NONE', *, *, #10800, .F. ) ;
#10220=CARTESIAN_POINT ( 'NONE',  ( -76.90625000000000000, 65.35533905932737753, -24.99999999999999645 ) ) ;
#10232=CARTESIAN_POINT ( 'NONE',  ( -72.87500000204839523, 65.69163855873949842, 25.81189881250000440 ) ) ;
#10239=CARTESIAN_POINT ( 'NONE',  ( -74.99999999999998579, 77.92805329443815765, -10.94505072500436604 ) ) ;
#10241=ORIENTED_EDGE ( 'NONE', *, *, #10800, .T. ) ;
#10244=CARTESIAN_POINT ( 'NONE',  ( -74.09375000409676204, 80.00000000000001421, -10.35533905932737753 ) ) ;
#10256=ADVANCED_FACE ( 'NONE', ( #2650 ), #4622, .F. ) ;
#10269=CARTESIAN_POINT ( 'NONE',  ( -78.03125000000002842, 79.99999999999992895, 10.35533905932734378 ) ) ;
#10277=CARTESIAN_POINT ( 'NONE',  ( -75.21875000000007105, 79.99999999999990052, -10.35533905932733312 ) ) ;
#10280=FACE_OUTER_BOUND ( 'NONE', #11678, .T. ) ;
#10281=CARTESIAN_POINT ( 'NONE',  ( -74.99999999999998579, 55.08591585515510047, -25.82567655465456724 ) ) ;
#10294=CARTESIAN_POINT ( 'NONE',  ( -72.96875000204838102, 73.25176868561975141, 18.25176868561974075 ) ) ;
#10302=CARTESIAN_POINT ( 'NONE',  ( -75.00000000000000000, 71.47984153822721964, -19.58526305464525308 ) ) ;
#10306=CARTESIAN_POINT ( 'NONE',  ( -74.28125000409676204, 65.35533905932737753, -24.99999999999999645 ) ) ;
#10335=CARTESIAN_POINT ( 'NONE',  ( -78.96875000000001421, 30.00000000000003908, 10.35533905932737753 ) ) ;
#10341=CARTESIAN_POINT ( 'NONE',  ( -74.93750000000000000, 72.67766952966368876, 17.67766952966368521 ) ) ;
#10355=CARTESIAN_POINT ( 'NONE',  ( -77.28125000204839523, 73.25176868561975141, 18.25176868561974075 ) ) ;
#10369=DIRECTION ( 'NONE',  ( -1.000000000000000000, 0.000000000000000000, 0.000000000000000000 ) ) ;
#10372=ADVANCED_FACE ( 'NONE', ( #6376 ), #1686, .F. ) ;
#10377=CARTESIAN_POINT ( 'NONE',  ( -79.43750000000004263, 72.67766952966367455, 17.67766952966366745 ) ) ;
#10397=CARTESIAN_POINT ( 'NONE',  ( -75.78125000000001421, 30.00000000000000355, -10.35533905932738108 ) ) ;
#10412=CARTESIAN_POINT ( 'NONE',  ( -72.12500000204839523, 44.30836144126050158, -25.81189881249999374 ) ) ;
#10423=CARTESIAN_POINT ( 'NONE',  ( -73.06250000409677625, 37.32233047033631124, -17.67766952966368166 ) ) ;
#10424=CARTESIAN_POINT ( 'NONE',  ( -75.00000000000000000, 55.00000000000000000, 0.000000000000000000 ) ) ;
#10432=ORIENTED_EDGE ( 'NONE', *, *, #4332, .F. ) ;
#10439=VERTEX_POINT ( 'NONE', #5712 ) ;
#10452=CARTESIAN_POINT ( 'NONE',  ( -78.03124999999998579, 80.00000000000001421, 10.35533905932737397 ) ) ;
#10466=CARTESIAN_POINT ( 'NONE',  ( -72.12500000204840944, 29.18810118750000626, -10.69163855873949309 ) ) ;
#10481=CARTESIAN_POINT ( 'NONE',  ( -71.18750000409677625, 72.67766952966368876, -17.67766952966368876 ) ) ;
#10484=ORIENTED_EDGE ( 'NONE', *, *, #3354, .T. ) ;
#10496=CIRCLE ( 'NONE', #7081, 20.00000000000000355 ) ;
#10508=( NAMED_UNIT ( * ) PLANE_ANGLE_UNIT ( ) SI_UNIT ( $, .RADIAN. ) );
#10512=CARTESIAN_POINT ( 'NONE',  ( -78.87500000204838102, 65.69163855873949842, 25.81189881250000440 ) ) ;
#10524=CARTESIAN_POINT ( 'NONE',  ( -75.96875000204839523, 80.81189881250000440, -1.580522963032174394E-15 ) ) ;
#10539=CARTESIAN_POINT ( 'NONE',  ( -79.43750000204838102, 55.00000000000000000, -24.99999999999999645 ) ) ;
#10550=DIRECTION ( 'NONE',  ( 0.000000000000000000, 0.000000000000000000, 1.000000000000000000 ) ) ;
#10557=CARTESIAN_POINT ( 'NONE',  ( -73.43750000204839523, 44.30836144126050158, -25.81189881249999374 ) ) ;
#10561=CARTESIAN_POINT ( 'NONE',  ( -75.00000000000001421, 34.09894944383669468, 14.06340364766198725 ) ) ;
#10571=CARTESIAN_POINT ( 'NONE',  ( -71.91717626682689968, 72.42551787026226862, 19.81812247078860523 ) ) ;
#10583=CARTESIAN_POINT ( 'NONE',  ( -74.46875000204839523, 80.81189881250000440, -1.580522963032174394E-15 ) ) ;
#10589=CARTESIAN_POINT ( 'NONE',  ( -77.93750000204838102, 65.69163855873948421, -25.81189881250000084 ) ) ;
#10601=CARTESIAN_POINT ( 'NONE',  ( -77.28125000000004263, 30.00000000000009948, -10.35533905932734378 ) ) ;
#10605=CARTESIAN_POINT ( 'NONE',  ( -77.28125000204839523, 73.25176868561975141, 18.25176868561974075 ) ) ;
#10606=EDGE_CURVE ( 'NONE', #2912, #9864, #7809, .T. ) ;
#10613=CARTESIAN_POINT ( 'NONE',  ( -75.00000000000001421, 42.56479188213557308, 21.68791366326873060 ) ) ;
#10616=ORIENTED_EDGE ( 'NONE', *, *, #9968, .T. ) ;
#10622=CARTESIAN_POINT ( 'NONE',  ( -79.53125000204838102, 55.00000000000000000, -25.81189881249999729 ) ) ;
#10635=CARTESIAN_POINT ( 'NONE',  ( -76.43750000204839523, 44.30836144126050158, -25.81189881249999374 ) ) ;
#10643=CARTESIAN_POINT ( 'NONE',  ( -76.25000000204838102, 80.81189881250000440, -10.69163855873948954 ) ) ;
#10660=CARTESIAN_POINT ( 'NONE',  ( -78.21875000409677625, 65.35533905932734910, 25.00000000000002132 ) ) ;
#10667=CARTESIAN_POINT ( 'NONE',  ( -79.15625000204839523, 73.25176868561975141, -18.25176868561974430 ) ) ;
#10672=CARTESIAN_POINT ( 'NONE',  ( -74.99999999999995737, 39.06450503476944647, 19.38126819931413181 ) ) ;
#10686=CARTESIAN_POINT ( 'NONE',  ( -78.78125000204838102, 55.00000000000000000, 25.81189881249999729 ) ) ;
#10690=CARTESIAN_POINT ( 'NONE',  ( -83.00000000000000000, 55.00000000000000000, -20.00000000000000355 ) ) ;
#10699=CYLINDRICAL_SURFACE ( 'NONE', #924, 25.00000000000000355 ) ;
#10700=CARTESIAN_POINT ( 'NONE',  ( -71.46875000204838102, 80.81189881250000440, -1.580522963032174394E-15 ) ) ;
#10718=ORIENTED_EDGE ( 'NONE', *, *, #1485, .T. ) ;
#10729=CARTESIAN_POINT ( 'NONE',  ( -78.31250000204839523, 29.18810118750000981, 10.69163855873950020 ) ) ;
#10735=CARTESIAN_POINT ( 'NONE',  ( -75.00000000000001421, 41.64360328783618570, 21.18013987092516359 ) ) ;
#10745=CARTESIAN_POINT ( 'NONE',  ( -77.00000000204838102, 29.18810118750000981, 10.69163855873950020 ) ) ;
#10785=CARTESIAN_POINT ( 'NONE',  ( -74.09375000204839523, 55.00000000000000000, 25.81189881249999729 ) ) ;
#10788=CARTESIAN_POINT ( 'NONE',  ( -77.09375000409677625, 80.00000000000001421, -10.35533905932737753 ) ) ;
#10791=CARTESIAN_POINT ( 'NONE',  ( -74.99999999999998579, 32.59534436559583526, -12.65407985245519917 ) ) ;
#10800=EDGE_CURVE ( 'NONE', #11066, #11373, #4559, .T. ) ;
#10801=CARTESIAN_POINT ( 'NONE',  ( -71.59560441993426139, 80.81189881250000440, 6.916273537586018705 ) ) ;
#10814=DIRECTION ( 'NONE',  ( -1.000000000000000000, 0.000000000000000000, 0.000000000000000000 ) ) ;
#10816=ORIENTED_EDGE ( 'NONE', *, *, #1799, .F. ) ;
#10832=CARTESIAN_POINT ( 'NONE',  ( -77.93750000204838102, 65.69163855873948421, -25.81189881250000440 ) ) ;
#10833=VERTEX_POINT ( 'NONE', #10944 ) ;
#10840=CARTESIAN_POINT ( 'NONE',  ( -78.21875000204839523, 29.18810118750000271, 4.741568889096522788E-15 ) ) ;
#10845=COLOUR_RGB ( '',0.8941176470588234615, 0.8941176470588234615, 0.8941176470588234615 ) ;
#10849=CARTESIAN_POINT ( 'NONE',  ( -76.15625000409677625, 30.00000000000000355, -10.35533905932738108 ) ) ;
#10861=ORIENTED_EDGE ( 'NONE', *, *, #8165, .F. ) ;
#10862=CARTESIAN_POINT ( 'NONE',  ( -76.71875000000004263, 79.99999999999990052, -10.35533905932733667 ) ) ;
#10872=DIRECTION ( 'NONE',  ( -1.000000000000000000, 0.000000000000000000, 0.000000000000000000 ) ) ;
#10892=CARTESIAN_POINT ( 'NONE',  ( -78.03125000204838102, 55.00000000000000000, -25.81189881249999729 ) ) ;
#10899=CARTESIAN_POINT ( 'NONE',  ( -77.37500000204838102, 80.81189881250000440, 10.69163855873948243 ) ) ;
#10907=CARTESIAN_POINT ( 'NONE',  ( -72.31250000204839523, 29.18810118750000981, 10.69163855873950020 ) ) ;
#10924=CARTESIAN_POINT ( 'NONE',  ( -71.44842626887532333, 72.99142816090481745, 20.46173487478911568 ) ) ;
#10943=VERTEX_POINT ( 'NONE', #2579 ) ;
#10944=CARTESIAN_POINT ( 'NONE',  ( -77.37500000409677625, 55.00000000000000000, -24.99999999999999645 ) ) ;
#10948=CARTESIAN_POINT ( 'NONE',  ( -76.81250000204838102, 29.18810118750000626, -10.69163855873949309 ) ) ;
#10949=ORIENTED_EDGE ( 'NONE', *, *, #913, .F. ) ;
#10954=CARTESIAN_POINT ( 'NONE',  ( -75.31250000204839523, 29.18810118750000981, 10.69163855873950020 ) ) ;
#10960=CARTESIAN_POINT ( 'NONE',  ( -72.87500000204840944, 80.81189881250001861, 10.69163855873948599 ) ) ;
#10973=CARTESIAN_POINT ( 'NONE',  ( -76.25000000204838102, 80.81189881250001861, -10.69163855873949132 ) ) ;
#10985=CARTESIAN_POINT ( 'NONE',  ( -75.00000000000000000, 55.00000000000000000, 0.000000000000000000 ) ) ;
#10986=CARTESIAN_POINT ( 'NONE',  ( -75.00000000000000000, 55.00000000000000000, -25.00000000000000355 ) ) ;
#11000=CARTESIAN_POINT ( 'NONE',  ( -78.40625000204838102, 29.18810118750000271, 4.741568889096522788E-15 ) ) ;
#11001=AXIS2_PLACEMENT_3D ( 'NONE', #6111, #5208, #4121 ) ;
#11008=CARTESIAN_POINT ( 'NONE',  ( -77.28125000204839523, 73.25176868561975141, 18.25176868561974075 ) ) ;
#11014=CARTESIAN_POINT ( 'NONE',  ( -77.18750000409679046, 72.67766952966368876, -17.67766952966368876 ) ) ;
#11039=AXIS2_PLACEMENT_3D ( 'NONE', #9113, #5523, #9171 ) ;
#11046=DIRECTION ( 'NONE',  ( -1.000000000000000000, 0.000000000000000000, 0.000000000000000000 ) ) ;
#11065=CARTESIAN_POINT ( 'NONE',  ( -75.96875000204839523, 73.25176868561975141, 18.25176868561974075 ) ) ;
#11066=VERTEX_POINT ( 'NONE', #823 ) ;
#11068=CIRCLE ( 'NONE', #7459, 25.00000000000000355 ) ;
#11073=CARTESIAN_POINT ( 'NONE',  ( -76.06250000204842365, 80.81189881250000440, -10.69163855873948954 ) ) ;
#11080=CARTESIAN_POINT ( 'NONE',  ( -71.93750000204838102, 44.30836144126050158, -25.81189881249999374 ) ) ;
#11081=CARTESIAN_POINT ( 'NONE',  ( -75.00000000000000000, 55.00000000000000000, -25.00000000000000355 ) ) ;
#11085=CARTESIAN_POINT ( 'NONE',  ( -75.00000000000000000, 55.00000000000000000, 0.000000000000000000 ) ) ;
#11110=CARTESIAN_POINT ( 'NONE',  ( -77.93750000000000000, 72.67766952966368876, 17.67766952966368521 ) ) ;
#11125=CARTESIAN_POINT ( 'NONE',  ( -73.53125000204838102, 55.00000000000000000, -25.81189881249999729 ) ) ;
#11132=DIRECTION ( 'NONE',  ( -1.000000000000000000, 0.000000000000000000, 0.000000000000000000 ) ) ;
#11136=CARTESIAN_POINT ( 'NONE',  ( -71.84375000409677625, 30.00000000000001421, 10.35533905932739174 ) ) ;
#11165=CARTESIAN_POINT ( 'NONE',  ( -77.56250000000000000, 37.32233047033631124, 17.67766952966369232 ) ) ;
#11180=CARTESIAN_POINT ( 'NONE',  ( -78.96875000204839523, 80.81189881250000440, -1.580522963032174394E-15 ) ) ;
#11189=( BOUNDED_CURVE ( )  B_SPLINE_CURVE ( 2, ( #3508, #2735, #3568, #10862, #2672, #3799, #7642, #6631, #5848 ),
 .UNSPECIFIED., .F., .T. ) 
 B_SPLINE_CURVE_WITH_KNOTS ( ( 3, 2, 2, 2, 3 ),
 ( 0.3168733201082642448, 0.3366713418703649596, 0.3564693636324655635, 0.3762673853945661673, 0.3960654071566668821 ),
 .UNSPECIFIED. ) 
 CURVE ( )  GEOMETRIC_REPRESENTATION_ITEM ( )  RATIONAL_B_SPLINE_CURVE ( ( 1.000000000000000000, 0.9238795325112868495, 1.000000000000000000, 0.9238795325112868495, 1.000000000000000000, 0.9238795325112868495, 1.000000000000000000, 0.9238795325112868495, 1.000000000000000000 ) ) 
 REPRESENTATION_ITEM ( '' )  );
#11198=CARTESIAN_POINT ( 'NONE',  ( -70.93935441986300816, 80.00000000000001421, 6.698726263377743351 ) ) ;
#11222=ORIENTED_EDGE ( 'NONE', *, *, #3731, .T. ) ;
#11229=CARTESIAN_POINT ( 'NONE',  ( -75.68750000409677625, 72.67766952966368876, -17.67766952966368876 ) ) ;
#11231=CARTESIAN_POINT ( 'NONE',  ( -76.25000000000000000, 55.00000000000000000, 24.99999999999999645 ) ) ;
#11243=CARTESIAN_POINT ( 'NONE',  ( -77.56250000204839523, 80.81189881250001861, -10.69163855873949132 ) ) ;
#11252=CARTESIAN_POINT ( 'NONE',  ( -75.00000000000004263, 59.49947659938870714, -25.42130211060962353 ) ) ;
#11257=CARTESIAN_POINT ( 'NONE',  ( -74.46875000409679046, 44.64466094067260826, -24.99999999999998934 ) ) ;
#11287=FACE_OUTER_BOUND ( 'NONE', #8246, .T. ) ;
#11288=CARTESIAN_POINT ( 'NONE',  ( -77.75000000409677625, 30.00000000000000355, 4.592425496802573578E-15 ) ) ;
#11293=CARTESIAN_POINT ( 'NONE',  ( -77.18750000000000000, 37.32233047033631124, -17.67766952966368166 ) ) ;
#11307=CARTESIAN_POINT ( 'NONE',  ( -73.62500000204839523, 44.30836144126050158, -25.81189881249999374 ) ) ;
#11314=CLOSED_SHELL ( 'NONE', ( #2940, #9711, #4843, #8700, #5662, #1306, #2097, #1819, #7178, #9306, #9894, #629, #4341, #4111, #10256, #6314, #7712, #5957, #10372 ) ) ;
#11315=CARTESIAN_POINT ( 'NONE',  ( -78.50000000204842365, 29.18810118750000981, 10.69163855873950020 ) ) ;
#11320=CARTESIAN_POINT ( 'NONE',  ( -70.87427368927673399, 76.65063840437987608, 12.49999426731031527 ) ) ;
#11350=CARTESIAN_POINT ( 'NONE',  ( -78.96875000000000000, 30.00000000000001421, 10.35533905932739174 ) ) ;
#11351=CARTESIAN_POINT ( 'NONE',  ( -74.99999999999997158, 43.66642528933169132, -23.23653603557184155 ) ) ;
#11352=AXIS2_PLACEMENT_3D ( 'NONE', #5384, #11046, #7483 ) ;
#11356=EDGE_LOOP ( 'NONE', ( #11825, #2761, #10949, #3764 ) ) ;
#11363=CARTESIAN_POINT ( 'NONE',  ( -73.43750000204839523, 65.69163855873948421, -25.81189881250000440 ) ) ;
#11364=ORIENTED_EDGE ( 'NONE', *, *, #1668, .T. ) ;
#11367=( LENGTH_UNIT ( ) NAMED_UNIT ( * ) SI_UNIT ( .MILLI., .METRE. ) );
#11373=VERTEX_POINT ( 'NONE', #6478 ) ;
#11402=CARTESIAN_POINT ( 'NONE',  ( -79.34375000204839523, 73.25176868561975141, -18.25176868561974430 ) ) ;
#11403=CARTESIAN_POINT ( 'NONE',  ( -74.99999999999998579, 45.21990583575040290, -23.90237970175139637 ) ) ;
#11417=CARTESIAN_POINT ( 'NONE',  ( -76.53125000204839523, 36.74823131438024859, -18.25176868561973720 ) ) ;
#11436=DIRECTION ( 'NONE',  ( 0.000000000000000000, 0.000000000000000000, 1.000000000000000000 ) ) ;
#11439=DIRECTION ( 'NONE',  ( 0.000000000000000000, 0.000000000000000000, 1.000000000000000000 ) ) ;
#11452=CARTESIAN_POINT ( 'NONE',  ( -75.00000000000000000, 38.26481293166236242, 18.71712631840276941 ) ) ;
#11461=( NAMED_UNIT ( * ) SI_UNIT ( $, .STERADIAN. ) SOLID_ANGLE_UNIT ( ) );
#11464=CARTESIAN_POINT ( 'NONE',  ( -72.06435441788588037, 80.00000000000001421, 6.698726029249594482 ) ) ;
#11476=CARTESIAN_POINT ( 'NONE',  ( -73.43750000204839523, 44.30836144126050158, -25.81189881249999374 ) ) ;
#11484=CIRCLE ( 'NONE', #6347, 25.00000000000000355 ) ;
#11485=CARTESIAN_POINT ( 'NONE',  ( -76.34375000204839523, 73.25176868561975141, -18.25176868561974430 ) ) ;
#11488=B_SPLINE_CURVE_WITH_KNOTS ( 'NONE', 3,
 ( #3260, #10735, #8957, #10672, #11452, #1579, #3500, #7166, #790, #10561, #4406, #1633, #4345, #8776, #5129, #2361, #9785, #11514, #9902, #730, #5246, #7997, #2486, #2543, #3439, #1697, #8893, #6033, #9668, #10791, #1466, #11631, #674, #618, #557, #4221 ),
 .UNSPECIFIED., .F., .F.,
 ( 4, 2, 2, 2, 2, 2, 2, 2, 2, 2, 2, 2, 2, 2, 2, 2, 2, 4 ),
 ( 2.099783704812584100E-15, 0.003153077943881680070, 0.006306155887761260258, 0.009459233831640840445, 0.01103577280358064051, 0.01261231177552044232, 0.01576538971940004766, 0.01734192869133985293, 0.01891846766327966167, 0.02522462355103887582, 0.02837770149491848290, 0.03153077943879808998, 0.03468385738267770052, 0.03626039635461750926, 0.03783693532655729719, 0.04414309121431648358, 0.04729616915819608719, 0.05044924710207567692 ),
 .UNSPECIFIED. ) ;
#11494=DIRECTION ( 'NONE',  ( 0.000000000000000000, 0.000000000000000000, 1.000000000000000000 ) ) ;
#11502=CARTESIAN_POINT ( 'NONE',  ( -77.56250000000007105, 37.32233047033638229, 17.67766952966362837 ) ) ;
#11509=CARTESIAN_POINT ( 'NONE',  ( -77.46875000204839523, 80.81189881250000440, -1.580522963032174394E-15 ) ) ;
#11514=CARTESIAN_POINT ( 'NONE',  ( -75.00000000000002842, 30.18774035812622714, 5.570907983300552146 ) ) ;
#11524=CARTESIAN_POINT ( 'NONE',  ( -78.03125000204838102, 55.00000000000000000, -25.81189881249999729 ) ) ;
#11537=CARTESIAN_POINT ( 'NONE',  ( -72.21875000204838102, 29.18810118750000271, 4.741568889096522788E-15 ) ) ;
#11544=CARTESIAN_POINT ( 'NONE',  ( -77.37500000204838102, 65.69163855873949842, 25.81189881250000084 ) ) ;
#11555=PRODUCT_DEFINITION_CONTEXT ( 'detailed design', #1636, 'design' ) ;
#11566=CARTESIAN_POINT ( 'NONE',  ( -78.21875000204839523, 29.18810118750000271, 4.741568889096522788E-15 ) ) ;
#11584=CARTESIAN_POINT ( 'NONE',  ( -73.43750000000000000, 72.67766952966368876, 17.67766952966368521 ) ) ;
#11596=CARTESIAN_POINT ( 'NONE',  ( -72.96875000204838102, 80.81189881250000440, -1.580522963032174394E-15 ) ) ;
#11605=CARTESIAN_POINT ( 'NONE',  ( -75.12500000204838102, 44.30836144126049447, -25.81189881249999019 ) ) ;
#11627=CARTESIAN_POINT ( 'NONE',  ( -74.37500000204838102, 80.81189881250001861, 10.69163855873948599 ) ) ;
#11631=CARTESIAN_POINT ( 'NONE',  ( -75.00000000000004263, 35.59195408377532743, -16.92649842553838724 ) ) ;
#11635=B_SPLINE_CURVE_WITH_KNOTS ( 'NONE', 1,
 ( #4885, #7757 ),
 .UNSPECIFIED., .F., .F.,
 ( 2, 2 ),
 ( 0.000000000000000000, 1.000000000000000000 ),
 .UNSPECIFIED. ) ;
#11643=CARTESIAN_POINT ( 'NONE',  ( -72.87500000000000000, 30.00000000000000355, 4.592425496802573578E-15 ) ) ;
#11645=EDGE_CURVE ( 'NONE', #879, #2912, #2196, .T. ) ;
#11651=CARTESIAN_POINT ( 'NONE',  ( -79.81250000000004263, 72.67766952966367455, -17.67766952966367100 ) ) ;
#11659=CARTESIAN_POINT ( 'NONE',  ( -75.78125000204839523, 73.25176868561975141, 18.25176868561974075 ) ) ;
#11664=VECTOR ( 'NONE', #1891, 1000.000000000000000 ) ;
#11670=DIRECTION ( 'NONE',  ( -1.000000000000000000, 0.000000000000000000, 0.000000000000000000 ) ) ;
#11678=EDGE_LOOP ( 'NONE', ( #7266, #83, #5088, #870, #8710, #5735, #2490, #3126, #2476, #5059 ) ) ;
#11683=DIRECTION ( 'NONE',  ( 1.000000000000000000, -0.000000000000000000, -0.000000000000000000 ) ) ;
#11691=CARTESIAN_POINT ( 'NONE',  ( -74.75000000204840944, 65.69163855873948421, -25.81189881250000440 ) ) ;
#11696=CARTESIAN_POINT ( 'NONE',  ( -76.81250000409679046, 72.67766952966368876, 17.67766952966368521 ) ) ;
#11708=CARTESIAN_POINT ( 'NONE',  ( -76.53125000204838102, 55.00000000000000000, -25.81189881249999729 ) ) ;
#11711=CARTESIAN_POINT ( 'NONE',  ( -79.53125000204838102, 55.00000000000000000, -25.81189881249999729 ) ) ;
#11722=( BOUNDED_CURVE ( )  B_SPLINE_CURVE ( 2, ( #4920, #2270, #5826, #8746, #5945, #3058, #8572, #4192, #529 ),
 .UNSPECIFIED., .F., .T. ) 
 B_SPLINE_CURVE_WITH_KNOTS ( ( 3, 2, 2, 2, 3 ),
 ( 0.3960654071566668821, 0.4158759072859810613, 0.4356864074152952404, 0.4554969075446094751, 0.4753074076739236542 ),
 .UNSPECIFIED. ) 
 CURVE ( )  GEOMETRIC_REPRESENTATION_ITEM ( )  RATIONAL_B_SPLINE_CURVE ( ( 1.000000000000000000, 0.9238795325112867385, 1.000000000000000000, 0.9238795325112867385, 1.000000000000000000, 0.9238795325112867385, 1.000000000000000000, 0.9238795325111756052, 1.000000000000111244 ) ) 
 REPRESENTATION_ITEM ( '' )  );
#11735=CARTESIAN_POINT ( 'NONE',  ( -79.25000000204838102, 80.81189881250001861, -10.69163855873949132 ) ) ;
#11741=CARTESIAN_POINT ( 'NONE',  ( -78.78125000204839523, 73.25176868561975141, 18.25176868561974075 ) ) ;
#11746=CARTESIAN_POINT ( 'NONE',  ( -75.87500000204839523, 80.81189881250001861, 10.69163855873948599 ) ) ;
#11751=ORIENTED_EDGE ( 'NONE', *, *, #4225, .T. ) ;
#11761=CARTESIAN_POINT ( 'NONE',  ( -71.65625000204838102, 80.81189881250000440, -1.580522963032174394E-15 ) ) ;
#11783=ORIENTED_EDGE ( 'NONE', *, *, #1485, .F. ) ;
#11790=CARTESIAN_POINT ( 'NONE',  ( -78.78125000204838102, 55.00000000000000000, 25.81189881249999729 ) ) ;
#11799=CARTESIAN_POINT ( 'NONE',  ( -75.59375000204839523, 55.00000000000000000, 25.81189881249999729 ) ) ;
#11802=AXIS2_PLACEMENT_3D ( 'NONE', #2258, #2202, #5814 ) ;
#11805=CARTESIAN_POINT ( 'NONE',  ( -76.25000000409677625, 30.00000000000000355, 4.592425496802573578E-15 ) ) ;
#11806=CARTESIAN_POINT ( 'NONE',  ( -75.31250000409677625, 72.67766952966368876, 17.67766952966368521 ) ) ;
#11808=DIRECTION ( 'NONE',  ( -1.000000000000000000, 0.000000000000000000, 0.000000000000000000 ) ) ;
#11818=ORIENTED_EDGE ( 'NONE', *, *, #5965, .T. ) ;
#11819=CARTESIAN_POINT ( 'NONE',  ( -73.90625000204838102, 29.18810118750000271, 4.741568889096522788E-15 ) ) ;
#11825=ORIENTED_EDGE ( 'NONE', *, *, #55, .T. ) ;
#11844=CARTESIAN_POINT ( 'NONE',  ( -76.53125000204838102, 55.00000000000000000, -25.81189881249999729 ) ) ;
#11868=COLOUR_RGB('Light Blue',0.38,0.62,0.78);
#11869=FILL_AREA_STYLE_COLOUR('',#11868);
#11870=FILL_AREA_STYLE('',(#11869));
#11871=SURFACE_STYLE_FILL_AREA(#11870);
#11872=SURFACE_SIDE_STYLE('',(#11871));
#11873=SURFACE_STYLE_USAGE(.BOTH.,#11872);
#11874=PRESENTATION_STYLE_ASSIGNMENT((#11873));
ENDSEC;
END-ISO-10303-21;
